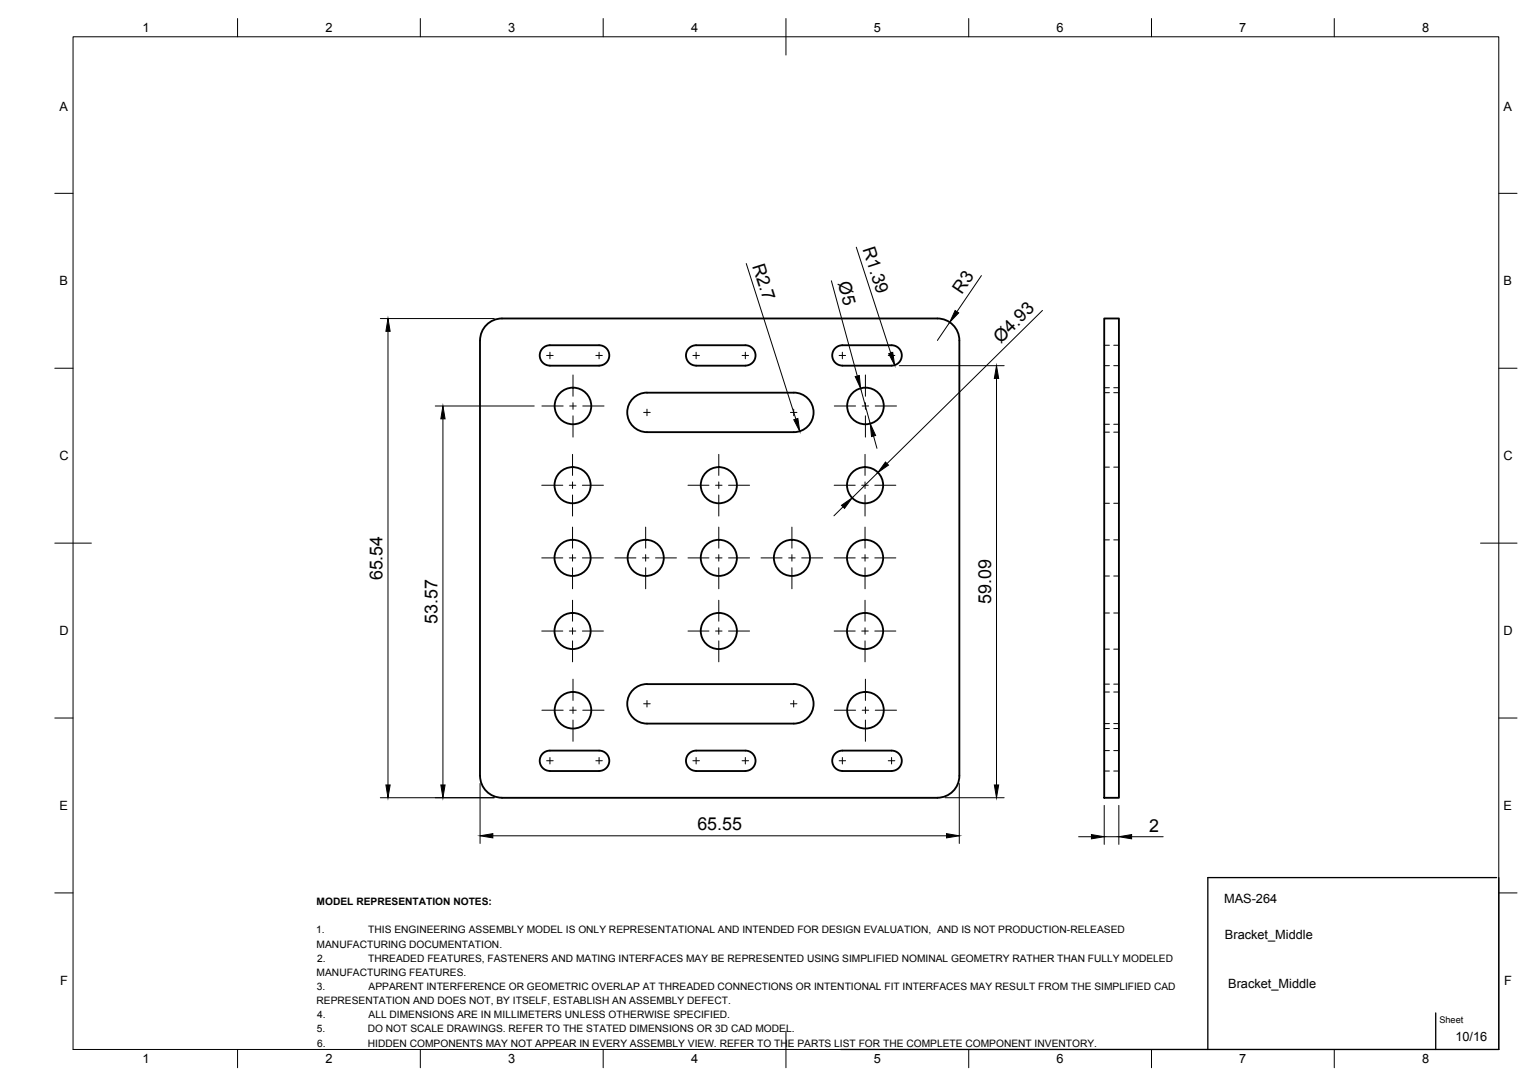
ISO-10303-21;
HEADER;
/* Generated by software containing ST-Developer
 * from STEP Tools, Inc. (www.steptools.com) 
 */

FILE_DESCRIPTION(
/* description */ (''),
/* implementation_level */ '2;1');

FILE_NAME(
/* name */ 'Bracket_Middle.step',
/* time_stamp */ '2026-10-12T15:37:13-07:00',
/* author */ (''),
/* organization */ (''),
/* preprocessor_version */ 'ST-DEVELOPER v20.2',
/* originating_system */ 'Autodesk Translation Framework v15.15.0.0',
/* authorisation */ '');

FILE_SCHEMA (('AUTOMOTIVE_DESIGN { 1 0 10303 214 3 1 1 }'));
ENDSEC;

DATA;
#10=MECHANICAL_DESIGN_GEOMETRIC_PRESENTATION_REPRESENTATION('',(#355),#36460);
#116=SHAPE_REPRESENTATION_RELATIONSHIP('SRR','None',#36528,#129);
#129=ADVANCED_BREP_SHAPE_REPRESENTATION('',(#387),#36457);
#207=FACE_BOUND('',#2295,.T.);
#208=FACE_BOUND('',#2296,.T.);
#209=FACE_BOUND('',#2297,.T.);
#210=FACE_BOUND('',#2298,.T.);
#211=FACE_BOUND('',#2299,.T.);
#212=FACE_BOUND('',#2300,.T.);
#213=FACE_BOUND('',#2301,.T.);
#214=FACE_BOUND('',#2302,.T.);
#215=FACE_BOUND('',#2303,.T.);
#216=FACE_BOUND('',#2304,.T.);
#217=FACE_BOUND('',#2305,.T.);
#218=FACE_BOUND('',#2306,.T.);
#219=FACE_BOUND('',#2307,.T.);
#220=FACE_BOUND('',#2308,.T.);
#221=FACE_BOUND('',#2309,.T.);
#222=FACE_BOUND('',#2310,.T.);
#223=FACE_BOUND('',#2311,.T.);
#224=FACE_BOUND('',#2312,.T.);
#225=FACE_BOUND('',#2313,.T.);
#226=FACE_BOUND('',#2314,.T.);
#227=FACE_BOUND('',#2315,.T.);
#228=FACE_BOUND('',#2316,.T.);
#229=FACE_BOUND('',#2317,.T.);
#230=FACE_BOUND('',#2319,.T.);
#231=FACE_BOUND('',#2320,.T.);
#232=FACE_BOUND('',#2321,.T.);
#233=FACE_BOUND('',#2322,.T.);
#234=FACE_BOUND('',#2323,.T.);
#235=FACE_BOUND('',#2324,.T.);
#236=FACE_BOUND('',#2325,.T.);
#237=FACE_BOUND('',#2326,.T.);
#238=FACE_BOUND('',#2327,.T.);
#239=FACE_BOUND('',#2328,.T.);
#240=FACE_BOUND('',#2329,.T.);
#241=FACE_BOUND('',#2330,.T.);
#242=FACE_BOUND('',#2331,.T.);
#243=FACE_BOUND('',#2332,.T.);
#244=FACE_BOUND('',#2333,.T.);
#245=FACE_BOUND('',#2334,.T.);
#246=FACE_BOUND('',#2335,.T.);
#247=FACE_BOUND('',#2336,.T.);
#248=FACE_BOUND('',#2337,.T.);
#249=FACE_BOUND('',#2338,.T.);
#250=FACE_BOUND('',#2339,.T.);
#251=FACE_BOUND('',#2340,.T.);
#252=FACE_BOUND('',#2341,.T.);
#355=STYLED_ITEM('',(#36596),#387);
#387=MANIFOLD_SOLID_BREP('Body1',#11291);
#671=PLANE('',#12235);
#672=PLANE('',#12239);
#673=PLANE('',#12258);
#674=PLANE('',#12262);
#675=PLANE('',#12266);
#676=PLANE('',#12270);
#677=PLANE('',#12289);
#678=PLANE('',#12293);
#679=PLANE('',#12303);
#680=PLANE('',#12307);
#681=PLANE('',#12311);
#682=PLANE('',#12315);
#683=PLANE('',#12319);
#684=PLANE('',#12323);
#685=PLANE('',#12327);
#686=PLANE('',#12331);
#687=PLANE('',#12341);
#688=PLANE('',#12345);
#689=PLANE('',#12349);
#690=PLANE('',#12353);
#691=PLANE('',#12357);
#692=PLANE('',#12358);
#1550=FACE_OUTER_BOUND('',#2239,.T.);
#1551=FACE_OUTER_BOUND('',#2240,.T.);
#1552=FACE_OUTER_BOUND('',#2241,.T.);
#1553=FACE_OUTER_BOUND('',#2242,.T.);
#1554=FACE_OUTER_BOUND('',#2243,.T.);
#1555=FACE_OUTER_BOUND('',#2244,.T.);
#1556=FACE_OUTER_BOUND('',#2245,.T.);
#1557=FACE_OUTER_BOUND('',#2246,.T.);
#1558=FACE_OUTER_BOUND('',#2247,.T.);
#1559=FACE_OUTER_BOUND('',#2248,.T.);
#1560=FACE_OUTER_BOUND('',#2249,.T.);
#1561=FACE_OUTER_BOUND('',#2250,.T.);
#1562=FACE_OUTER_BOUND('',#2251,.T.);
#1563=FACE_OUTER_BOUND('',#2252,.T.);
#1564=FACE_OUTER_BOUND('',#2253,.T.);
#1565=FACE_OUTER_BOUND('',#2254,.T.);
#1566=FACE_OUTER_BOUND('',#2255,.T.);
#1567=FACE_OUTER_BOUND('',#2256,.T.);
#1568=FACE_OUTER_BOUND('',#2257,.T.);
#1569=FACE_OUTER_BOUND('',#2258,.T.);
#1570=FACE_OUTER_BOUND('',#2259,.T.);
#1571=FACE_OUTER_BOUND('',#2260,.T.);
#1572=FACE_OUTER_BOUND('',#2261,.T.);
#1573=FACE_OUTER_BOUND('',#2262,.T.);
#1574=FACE_OUTER_BOUND('',#2263,.T.);
#1575=FACE_OUTER_BOUND('',#2264,.T.);
#1576=FACE_OUTER_BOUND('',#2265,.T.);
#1577=FACE_OUTER_BOUND('',#2266,.T.);
#1578=FACE_OUTER_BOUND('',#2267,.T.);
#1579=FACE_OUTER_BOUND('',#2268,.T.);
#1580=FACE_OUTER_BOUND('',#2269,.T.);
#1581=FACE_OUTER_BOUND('',#2270,.T.);
#1582=FACE_OUTER_BOUND('',#2271,.T.);
#1583=FACE_OUTER_BOUND('',#2272,.T.);
#1584=FACE_OUTER_BOUND('',#2273,.T.);
#1585=FACE_OUTER_BOUND('',#2274,.T.);
#1586=FACE_OUTER_BOUND('',#2275,.T.);
#1587=FACE_OUTER_BOUND('',#2276,.T.);
#1588=FACE_OUTER_BOUND('',#2277,.T.);
#1589=FACE_OUTER_BOUND('',#2278,.T.);
#1590=FACE_OUTER_BOUND('',#2279,.T.);
#1591=FACE_OUTER_BOUND('',#2280,.T.);
#1592=FACE_OUTER_BOUND('',#2281,.T.);
#1593=FACE_OUTER_BOUND('',#2282,.T.);
#1594=FACE_OUTER_BOUND('',#2283,.T.);
#1595=FACE_OUTER_BOUND('',#2284,.T.);
#1596=FACE_OUTER_BOUND('',#2285,.T.);
#1597=FACE_OUTER_BOUND('',#2286,.T.);
#1598=FACE_OUTER_BOUND('',#2287,.T.);
#1599=FACE_OUTER_BOUND('',#2288,.T.);
#1600=FACE_OUTER_BOUND('',#2289,.T.);
#1601=FACE_OUTER_BOUND('',#2290,.T.);
#1602=FACE_OUTER_BOUND('',#2291,.T.);
#1603=FACE_OUTER_BOUND('',#2292,.T.);
#1604=FACE_OUTER_BOUND('',#2293,.T.);
#1605=FACE_OUTER_BOUND('',#2294,.T.);
#1606=FACE_OUTER_BOUND('',#2318,.T.);
#2239=EDGE_LOOP('',(#9938,#9939,#9940,#9941));
#2240=EDGE_LOOP('',(#9942,#9943,#9944,#9945));
#2241=EDGE_LOOP('',(#9946,#9947,#9948,#9949));
#2242=EDGE_LOOP('',(#9950,#9951,#9952,#9953));
#2243=EDGE_LOOP('',(#9954,#9955,#9956,#9957));
#2244=EDGE_LOOP('',(#9958,#9959,#9960,#9961));
#2245=EDGE_LOOP('',(#9962,#9963,#9964,#9965));
#2246=EDGE_LOOP('',(#9966,#9967,#9968,#9969));
#2247=EDGE_LOOP('',(#9970,#9971,#9972,#9973));
#2248=EDGE_LOOP('',(#9974,#9975,#9976,#9977));
#2249=EDGE_LOOP('',(#9978,#9979,#9980,#9981));
#2250=EDGE_LOOP('',(#9982,#9983,#9984,#9985));
#2251=EDGE_LOOP('',(#9986,#9987,#9988,#9989));
#2252=EDGE_LOOP('',(#9990,#9991,#9992,#9993));
#2253=EDGE_LOOP('',(#9994,#9995,#9996,#9997));
#2254=EDGE_LOOP('',(#9998,#9999,#10000,#10001));
#2255=EDGE_LOOP('',(#10002,#10003,#10004,#10005));
#2256=EDGE_LOOP('',(#10006,#10007,#10008,#10009));
#2257=EDGE_LOOP('',(#10010,#10011,#10012,#10013));
#2258=EDGE_LOOP('',(#10014,#10015,#10016,#10017));
#2259=EDGE_LOOP('',(#10018,#10019,#10020,#10021));
#2260=EDGE_LOOP('',(#10022,#10023,#10024,#10025));
#2261=EDGE_LOOP('',(#10026,#10027,#10028,#10029));
#2262=EDGE_LOOP('',(#10030,#10031,#10032,#10033));
#2263=EDGE_LOOP('',(#10034,#10035,#10036,#10037));
#2264=EDGE_LOOP('',(#10038,#10039,#10040,#10041));
#2265=EDGE_LOOP('',(#10042,#10043,#10044,#10045));
#2266=EDGE_LOOP('',(#10046,#10047,#10048,#10049));
#2267=EDGE_LOOP('',(#10050,#10051,#10052,#10053));
#2268=EDGE_LOOP('',(#10054,#10055,#10056,#10057));
#2269=EDGE_LOOP('',(#10058,#10059,#10060,#10061));
#2270=EDGE_LOOP('',(#10062,#10063,#10064,#10065));
#2271=EDGE_LOOP('',(#10066,#10067,#10068,#10069));
#2272=EDGE_LOOP('',(#10070,#10071,#10072,#10073));
#2273=EDGE_LOOP('',(#10074,#10075,#10076,#10077));
#2274=EDGE_LOOP('',(#10078,#10079,#10080,#10081));
#2275=EDGE_LOOP('',(#10082,#10083,#10084,#10085));
#2276=EDGE_LOOP('',(#10086,#10087,#10088,#10089));
#2277=EDGE_LOOP('',(#10090,#10091,#10092,#10093));
#2278=EDGE_LOOP('',(#10094,#10095,#10096,#10097));
#2279=EDGE_LOOP('',(#10098,#10099,#10100,#10101));
#2280=EDGE_LOOP('',(#10102,#10103,#10104,#10105));
#2281=EDGE_LOOP('',(#10106,#10107,#10108,#10109));
#2282=EDGE_LOOP('',(#10110,#10111,#10112,#10113));
#2283=EDGE_LOOP('',(#10114,#10115,#10116,#10117));
#2284=EDGE_LOOP('',(#10118,#10119,#10120,#10121));
#2285=EDGE_LOOP('',(#10122,#10123,#10124,#10125));
#2286=EDGE_LOOP('',(#10126,#10127,#10128,#10129));
#2287=EDGE_LOOP('',(#10130,#10131,#10132,#10133));
#2288=EDGE_LOOP('',(#10134,#10135,#10136,#10137));
#2289=EDGE_LOOP('',(#10138,#10139,#10140,#10141));
#2290=EDGE_LOOP('',(#10142,#10143,#10144,#10145));
#2291=EDGE_LOOP('',(#10146,#10147,#10148,#10149));
#2292=EDGE_LOOP('',(#10150,#10151,#10152,#10153));
#2293=EDGE_LOOP('',(#10154,#10155,#10156,#10157));
#2294=EDGE_LOOP('',(#10158,#10159,#10160,#10161,#10162,#10163,#10164,#10165));
#2295=EDGE_LOOP('',(#10166));
#2296=EDGE_LOOP('',(#10167));
#2297=EDGE_LOOP('',(#10168,#10169,#10170,#10171));
#2298=EDGE_LOOP('',(#10172,#10173,#10174,#10175));
#2299=EDGE_LOOP('',(#10176,#10177,#10178,#10179));
#2300=EDGE_LOOP('',(#10180,#10181,#10182,#10183));
#2301=EDGE_LOOP('',(#10184));
#2302=EDGE_LOOP('',(#10185));
#2303=EDGE_LOOP('',(#10186,#10187,#10188,#10189));
#2304=EDGE_LOOP('',(#10190));
#2305=EDGE_LOOP('',(#10191));
#2306=EDGE_LOOP('',(#10192));
#2307=EDGE_LOOP('',(#10193));
#2308=EDGE_LOOP('',(#10194));
#2309=EDGE_LOOP('',(#10195,#10196,#10197,#10198));
#2310=EDGE_LOOP('',(#10199,#10200,#10201,#10202));
#2311=EDGE_LOOP('',(#10203));
#2312=EDGE_LOOP('',(#10204));
#2313=EDGE_LOOP('',(#10205));
#2314=EDGE_LOOP('',(#10206));
#2315=EDGE_LOOP('',(#10207));
#2316=EDGE_LOOP('',(#10208,#10209,#10210,#10211));
#2317=EDGE_LOOP('',(#10212));
#2318=EDGE_LOOP('',(#10213,#10214,#10215,#10216,#10217,#10218,#10219,#10220));
#2319=EDGE_LOOP('',(#10221));
#2320=EDGE_LOOP('',(#10222));
#2321=EDGE_LOOP('',(#10223,#10224,#10225,#10226));
#2322=EDGE_LOOP('',(#10227,#10228,#10229,#10230));
#2323=EDGE_LOOP('',(#10231,#10232,#10233,#10234));
#2324=EDGE_LOOP('',(#10235,#10236,#10237,#10238));
#2325=EDGE_LOOP('',(#10239));
#2326=EDGE_LOOP('',(#10240));
#2327=EDGE_LOOP('',(#10241,#10242,#10243,#10244));
#2328=EDGE_LOOP('',(#10245));
#2329=EDGE_LOOP('',(#10246));
#2330=EDGE_LOOP('',(#10247));
#2331=EDGE_LOOP('',(#10248));
#2332=EDGE_LOOP('',(#10249));
#2333=EDGE_LOOP('',(#10250,#10251,#10252,#10253));
#2334=EDGE_LOOP('',(#10254,#10255,#10256,#10257));
#2335=EDGE_LOOP('',(#10258));
#2336=EDGE_LOOP('',(#10259));
#2337=EDGE_LOOP('',(#10260));
#2338=EDGE_LOOP('',(#10261));
#2339=EDGE_LOOP('',(#10262));
#2340=EDGE_LOOP('',(#10263,#10264,#10265,#10266));
#2341=EDGE_LOOP('',(#10267));
#3192=LINE('',#35931,#4138);
#3193=LINE('',#35936,#4139);
#3194=LINE('',#35938,#4140);
#3195=LINE('',#35940,#4141);
#3196=LINE('',#35941,#4142);
#3197=LINE('',#35947,#4143);
#3198=LINE('',#35950,#4144);
#3199=LINE('',#35952,#4145);
#3200=LINE('',#35953,#4146);
#3201=LINE('',#35961,#4147);
#3202=LINE('',#35967,#4148);
#3203=LINE('',#35973,#4149);
#3204=LINE('',#35979,#4150);
#3205=LINE('',#35985,#4151);
#3206=LINE('',#35990,#4152);
#3207=LINE('',#35992,#4153);
#3208=LINE('',#35994,#4154);
#3209=LINE('',#35995,#4155);
#3210=LINE('',#36001,#4156);
#3211=LINE('',#36004,#4157);
#3212=LINE('',#36006,#4158);
#3213=LINE('',#36007,#4159);
#3214=LINE('',#36014,#4160);
#3215=LINE('',#36016,#4161);
#3216=LINE('',#36018,#4162);
#3217=LINE('',#36019,#4163);
#3218=LINE('',#36025,#4164);
#3219=LINE('',#36028,#4165);
#3220=LINE('',#36030,#4166);
#3221=LINE('',#36031,#4167);
#3222=LINE('',#36039,#4168);
#3223=LINE('',#36045,#4169);
#3224=LINE('',#36051,#4170);
#3225=LINE('',#36057,#4171);
#3226=LINE('',#36063,#4172);
#3227=LINE('',#36068,#4173);
#3228=LINE('',#36070,#4174);
#3229=LINE('',#36072,#4175);
#3230=LINE('',#36073,#4176);
#3231=LINE('',#36079,#4177);
#3232=LINE('',#36082,#4178);
#3233=LINE('',#36084,#4179);
#3234=LINE('',#36085,#4180);
#3235=LINE('',#36093,#4181);
#3236=LINE('',#36099,#4182);
#3237=LINE('',#36104,#4183);
#3238=LINE('',#36106,#4184);
#3239=LINE('',#36108,#4185);
#3240=LINE('',#36109,#4186);
#3241=LINE('',#36115,#4187);
#3242=LINE('',#36118,#4188);
#3243=LINE('',#36120,#4189);
#3244=LINE('',#36121,#4190);
#3245=LINE('',#36128,#4191);
#3246=LINE('',#36130,#4192);
#3247=LINE('',#36132,#4193);
#3248=LINE('',#36133,#4194);
#3249=LINE('',#36139,#4195);
#3250=LINE('',#36142,#4196);
#3251=LINE('',#36144,#4197);
#3252=LINE('',#36145,#4198);
#3253=LINE('',#36152,#4199);
#3254=LINE('',#36154,#4200);
#3255=LINE('',#36156,#4201);
#3256=LINE('',#36157,#4202);
#3257=LINE('',#36163,#4203);
#3258=LINE('',#36166,#4204);
#3259=LINE('',#36168,#4205);
#3260=LINE('',#36169,#4206);
#3261=LINE('',#36176,#4207);
#3262=LINE('',#36178,#4208);
#3263=LINE('',#36180,#4209);
#3264=LINE('',#36181,#4210);
#3265=LINE('',#36187,#4211);
#3266=LINE('',#36190,#4212);
#3267=LINE('',#36192,#4213);
#3268=LINE('',#36193,#4214);
#3269=LINE('',#36201,#4215);
#3270=LINE('',#36207,#4216);
#3271=LINE('',#36212,#4217);
#3272=LINE('',#36214,#4218);
#3273=LINE('',#36216,#4219);
#3274=LINE('',#36217,#4220);
#3275=LINE('',#36223,#4221);
#3276=LINE('',#36226,#4222);
#3277=LINE('',#36228,#4223);
#3278=LINE('',#36229,#4224);
#3279=LINE('',#36235,#4225);
#3280=LINE('',#36238,#4226);
#3281=LINE('',#36240,#4227);
#3282=LINE('',#36241,#4228);
#3283=LINE('',#36247,#4229);
#3284=LINE('',#36250,#4230);
#3285=LINE('',#36252,#4231);
#3286=LINE('',#36253,#4232);
#4138=VECTOR('',#14833,2.5);
#4139=VECTOR('',#14838,10.);
#4140=VECTOR('',#14839,10.);
#4141=VECTOR('',#14840,10.);
#4142=VECTOR('',#14841,10.);
#4143=VECTOR('',#14848,10.);
#4144=VECTOR('',#14851,10.);
#4145=VECTOR('',#14852,10.);
#4146=VECTOR('',#14853,10.);
#4147=VECTOR('',#14864,2.46675107308807);
#4148=VECTOR('',#14871,2.46675107308807);
#4149=VECTOR('',#14878,2.46675107308807);
#4150=VECTOR('',#14885,2.46675107308807);
#4151=VECTOR('',#14892,2.46675107308807);
#4152=VECTOR('',#14897,10.);
#4153=VECTOR('',#14898,10.);
#4154=VECTOR('',#14899,10.);
#4155=VECTOR('',#14900,10.);
#4156=VECTOR('',#14907,10.);
#4157=VECTOR('',#14910,10.);
#4158=VECTOR('',#14911,10.);
#4159=VECTOR('',#14912,10.);
#4160=VECTOR('',#14921,10.);
#4161=VECTOR('',#14922,10.);
#4162=VECTOR('',#14923,10.);
#4163=VECTOR('',#14924,10.);
#4164=VECTOR('',#14931,10.);
#4165=VECTOR('',#14934,10.);
#4166=VECTOR('',#14935,10.);
#4167=VECTOR('',#14936,10.);
#4168=VECTOR('',#14947,2.5);
#4169=VECTOR('',#14954,2.46675107308807);
#4170=VECTOR('',#14961,2.5);
#4171=VECTOR('',#14968,2.46675107308807);
#4172=VECTOR('',#14975,2.46675107308807);
#4173=VECTOR('',#14980,10.);
#4174=VECTOR('',#14981,10.);
#4175=VECTOR('',#14982,10.);
#4176=VECTOR('',#14983,10.);
#4177=VECTOR('',#14990,10.);
#4178=VECTOR('',#14993,10.);
#4179=VECTOR('',#14994,10.);
#4180=VECTOR('',#14995,10.);
#4181=VECTOR('',#15006,2.5);
#4182=VECTOR('',#15013,2.46675107308807);
#4183=VECTOR('',#15018,10.);
#4184=VECTOR('',#15019,10.);
#4185=VECTOR('',#15020,10.);
#4186=VECTOR('',#15021,10.);
#4187=VECTOR('',#15028,10.);
#4188=VECTOR('',#15031,10.);
#4189=VECTOR('',#15032,10.);
#4190=VECTOR('',#15033,10.);
#4191=VECTOR('',#15042,10.);
#4192=VECTOR('',#15043,10.);
#4193=VECTOR('',#15044,10.);
#4194=VECTOR('',#15045,10.);
#4195=VECTOR('',#15052,10.);
#4196=VECTOR('',#15055,10.);
#4197=VECTOR('',#15056,10.);
#4198=VECTOR('',#15057,10.);
#4199=VECTOR('',#15066,10.);
#4200=VECTOR('',#15067,10.);
#4201=VECTOR('',#15068,10.);
#4202=VECTOR('',#15069,10.);
#4203=VECTOR('',#15076,10.);
#4204=VECTOR('',#15079,10.);
#4205=VECTOR('',#15080,10.);
#4206=VECTOR('',#15081,10.);
#4207=VECTOR('',#15090,10.);
#4208=VECTOR('',#15091,10.);
#4209=VECTOR('',#15092,10.);
#4210=VECTOR('',#15093,10.);
#4211=VECTOR('',#15100,10.);
#4212=VECTOR('',#15103,10.);
#4213=VECTOR('',#15104,10.);
#4214=VECTOR('',#15105,10.);
#4215=VECTOR('',#15116,2.46675107308807);
#4216=VECTOR('',#15123,2.46675107308807);
#4217=VECTOR('',#15128,10.);
#4218=VECTOR('',#15129,10.);
#4219=VECTOR('',#15130,10.);
#4220=VECTOR('',#15131,10.);
#4221=VECTOR('',#15138,10.);
#4222=VECTOR('',#15141,10.);
#4223=VECTOR('',#15142,10.);
#4224=VECTOR('',#15143,10.);
#4225=VECTOR('',#15150,10.);
#4226=VECTOR('',#15153,10.);
#4227=VECTOR('',#15154,10.);
#4228=VECTOR('',#15155,10.);
#4229=VECTOR('',#15162,10.);
#4230=VECTOR('',#15165,10.);
#4231=VECTOR('',#15166,10.);
#4232=VECTOR('',#15167,10.);
#4497=CIRCLE('',#12233,2.5);
#4498=CIRCLE('',#12234,2.5);
#4499=CIRCLE('',#12237,1.3925055570925);
#4500=CIRCLE('',#12238,1.3925055570925);
#4501=CIRCLE('',#12241,1.3925055570925);
#4502=CIRCLE('',#12242,1.3925055570925);
#4503=CIRCLE('',#12244,2.46675107308807);
#4504=CIRCLE('',#12245,2.46675107308807);
#4505=CIRCLE('',#12247,2.46675107308807);
#4506=CIRCLE('',#12248,2.46675107308807);
#4507=CIRCLE('',#12250,2.46675107308807);
#4508=CIRCLE('',#12251,2.46675107308807);
#4509=CIRCLE('',#12253,2.46675107308807);
#4510=CIRCLE('',#12254,2.46675107308807);
#4511=CIRCLE('',#12256,2.46675107308807);
#4512=CIRCLE('',#12257,2.46675107308807);
#4513=CIRCLE('',#12260,2.69990459756453);
#4514=CIRCLE('',#12261,2.69990459756453);
#4515=CIRCLE('',#12264,2.69990459756453);
#4516=CIRCLE('',#12265,2.69990459756453);
#4517=CIRCLE('',#12268,1.3925055570925);
#4518=CIRCLE('',#12269,1.3925055570925);
#4519=CIRCLE('',#12272,1.3925055570925);
#4520=CIRCLE('',#12273,1.3925055570925);
#4521=CIRCLE('',#12275,2.5);
#4522=CIRCLE('',#12276,2.5);
#4523=CIRCLE('',#12278,2.46675107308807);
#4524=CIRCLE('',#12279,2.46675107308807);
#4525=CIRCLE('',#12281,2.5);
#4526=CIRCLE('',#12282,2.5);
#4527=CIRCLE('',#12284,2.46675107308807);
#4528=CIRCLE('',#12285,2.46675107308807);
#4529=CIRCLE('',#12287,2.46675107308807);
#4530=CIRCLE('',#12288,2.46675107308807);
#4531=CIRCLE('',#12291,1.3925055570925);
#4532=CIRCLE('',#12292,1.3925055570925);
#4533=CIRCLE('',#12295,1.3925055570925);
#4534=CIRCLE('',#12296,1.3925055570925);
#4535=CIRCLE('',#12298,2.5);
#4536=CIRCLE('',#12299,2.5);
#4537=CIRCLE('',#12301,2.46675107308807);
#4538=CIRCLE('',#12302,2.46675107308807);
#4539=CIRCLE('',#12305,1.3925055570925);
#4540=CIRCLE('',#12306,1.3925055570925);
#4541=CIRCLE('',#12309,1.3925055570925);
#4542=CIRCLE('',#12310,1.3925055570925);
#4543=CIRCLE('',#12313,1.3925055570925);
#4544=CIRCLE('',#12314,1.3925055570925);
#4545=CIRCLE('',#12317,1.3925055570925);
#4546=CIRCLE('',#12318,1.3925055570925);
#4547=CIRCLE('',#12321,1.3925055570925);
#4548=CIRCLE('',#12322,1.3925055570925);
#4549=CIRCLE('',#12325,1.3925055570925);
#4550=CIRCLE('',#12326,1.3925055570925);
#4551=CIRCLE('',#12329,2.69990459756453);
#4552=CIRCLE('',#12330,2.69990459756453);
#4553=CIRCLE('',#12333,2.69990459756453);
#4554=CIRCLE('',#12334,2.69990459756453);
#4555=CIRCLE('',#12336,2.46675107308807);
#4556=CIRCLE('',#12337,2.46675107308807);
#4557=CIRCLE('',#12339,2.46675107308807);
#4558=CIRCLE('',#12340,2.46675107308807);
#4559=CIRCLE('',#12343,3.00000000000004);
#4560=CIRCLE('',#12344,3.00000000000004);
#4561=CIRCLE('',#12347,3.00000000000003);
#4562=CIRCLE('',#12348,3.00000000000003);
#4563=CIRCLE('',#12351,3.00000000000004);
#4564=CIRCLE('',#12352,3.00000000000004);
#4565=CIRCLE('',#12355,3.00000000000004);
#4566=CIRCLE('',#12356,3.00000000000004);
#5495=VERTEX_POINT('',#35928);
#5496=VERTEX_POINT('',#35930);
#5497=VERTEX_POINT('',#35934);
#5498=VERTEX_POINT('',#35935);
#5499=VERTEX_POINT('',#35937);
#5500=VERTEX_POINT('',#35939);
#5501=VERTEX_POINT('',#35943);
#5502=VERTEX_POINT('',#35945);
#5503=VERTEX_POINT('',#35949);
#5504=VERTEX_POINT('',#35951);
#5505=VERTEX_POINT('',#35958);
#5506=VERTEX_POINT('',#35960);
#5507=VERTEX_POINT('',#35964);
#5508=VERTEX_POINT('',#35966);
#5509=VERTEX_POINT('',#35970);
#5510=VERTEX_POINT('',#35972);
#5511=VERTEX_POINT('',#35976);
#5512=VERTEX_POINT('',#35978);
#5513=VERTEX_POINT('',#35982);
#5514=VERTEX_POINT('',#35984);
#5515=VERTEX_POINT('',#35988);
#5516=VERTEX_POINT('',#35989);
#5517=VERTEX_POINT('',#35991);
#5518=VERTEX_POINT('',#35993);
#5519=VERTEX_POINT('',#35997);
#5520=VERTEX_POINT('',#35999);
#5521=VERTEX_POINT('',#36003);
#5522=VERTEX_POINT('',#36005);
#5523=VERTEX_POINT('',#36012);
#5524=VERTEX_POINT('',#36013);
#5525=VERTEX_POINT('',#36015);
#5526=VERTEX_POINT('',#36017);
#5527=VERTEX_POINT('',#36021);
#5528=VERTEX_POINT('',#36023);
#5529=VERTEX_POINT('',#36027);
#5530=VERTEX_POINT('',#36029);
#5531=VERTEX_POINT('',#36036);
#5532=VERTEX_POINT('',#36038);
#5533=VERTEX_POINT('',#36042);
#5534=VERTEX_POINT('',#36044);
#5535=VERTEX_POINT('',#36048);
#5536=VERTEX_POINT('',#36050);
#5537=VERTEX_POINT('',#36054);
#5538=VERTEX_POINT('',#36056);
#5539=VERTEX_POINT('',#36060);
#5540=VERTEX_POINT('',#36062);
#5541=VERTEX_POINT('',#36066);
#5542=VERTEX_POINT('',#36067);
#5543=VERTEX_POINT('',#36069);
#5544=VERTEX_POINT('',#36071);
#5545=VERTEX_POINT('',#36075);
#5546=VERTEX_POINT('',#36077);
#5547=VERTEX_POINT('',#36081);
#5548=VERTEX_POINT('',#36083);
#5549=VERTEX_POINT('',#36090);
#5550=VERTEX_POINT('',#36092);
#5551=VERTEX_POINT('',#36096);
#5552=VERTEX_POINT('',#36098);
#5553=VERTEX_POINT('',#36102);
#5554=VERTEX_POINT('',#36103);
#5555=VERTEX_POINT('',#36105);
#5556=VERTEX_POINT('',#36107);
#5557=VERTEX_POINT('',#36111);
#5558=VERTEX_POINT('',#36113);
#5559=VERTEX_POINT('',#36117);
#5560=VERTEX_POINT('',#36119);
#5561=VERTEX_POINT('',#36126);
#5562=VERTEX_POINT('',#36127);
#5563=VERTEX_POINT('',#36129);
#5564=VERTEX_POINT('',#36131);
#5565=VERTEX_POINT('',#36135);
#5566=VERTEX_POINT('',#36137);
#5567=VERTEX_POINT('',#36141);
#5568=VERTEX_POINT('',#36143);
#5569=VERTEX_POINT('',#36150);
#5570=VERTEX_POINT('',#36151);
#5571=VERTEX_POINT('',#36153);
#5572=VERTEX_POINT('',#36155);
#5573=VERTEX_POINT('',#36159);
#5574=VERTEX_POINT('',#36161);
#5575=VERTEX_POINT('',#36165);
#5576=VERTEX_POINT('',#36167);
#5577=VERTEX_POINT('',#36174);
#5578=VERTEX_POINT('',#36175);
#5579=VERTEX_POINT('',#36177);
#5580=VERTEX_POINT('',#36179);
#5581=VERTEX_POINT('',#36183);
#5582=VERTEX_POINT('',#36185);
#5583=VERTEX_POINT('',#36189);
#5584=VERTEX_POINT('',#36191);
#5585=VERTEX_POINT('',#36198);
#5586=VERTEX_POINT('',#36200);
#5587=VERTEX_POINT('',#36204);
#5588=VERTEX_POINT('',#36206);
#5589=VERTEX_POINT('',#36210);
#5590=VERTEX_POINT('',#36211);
#5591=VERTEX_POINT('',#36213);
#5592=VERTEX_POINT('',#36215);
#5593=VERTEX_POINT('',#36219);
#5594=VERTEX_POINT('',#36221);
#5595=VERTEX_POINT('',#36225);
#5596=VERTEX_POINT('',#36227);
#5597=VERTEX_POINT('',#36231);
#5598=VERTEX_POINT('',#36233);
#5599=VERTEX_POINT('',#36237);
#5600=VERTEX_POINT('',#36239);
#5601=VERTEX_POINT('',#36243);
#5602=VERTEX_POINT('',#36245);
#5603=VERTEX_POINT('',#36249);
#5604=VERTEX_POINT('',#36251);
#7000=EDGE_CURVE('',#5495,#5495,#4497,.T.);
#7001=EDGE_CURVE('',#5495,#5496,#3192,.T.);
#7002=EDGE_CURVE('',#5496,#5496,#4498,.T.);
#7003=EDGE_CURVE('',#5497,#5498,#3193,.T.);
#7004=EDGE_CURVE('',#5498,#5499,#3194,.T.);
#7005=EDGE_CURVE('',#5500,#5499,#3195,.T.);
#7006=EDGE_CURVE('',#5497,#5500,#3196,.T.);
#7007=EDGE_CURVE('',#5501,#5497,#4499,.T.);
#7008=EDGE_CURVE('',#5502,#5500,#4500,.T.);
#7009=EDGE_CURVE('',#5501,#5502,#3197,.T.);
#7010=EDGE_CURVE('',#5503,#5501,#3198,.T.);
#7011=EDGE_CURVE('',#5504,#5502,#3199,.T.);
#7012=EDGE_CURVE('',#5503,#5504,#3200,.T.);
#7013=EDGE_CURVE('',#5498,#5503,#4501,.T.);
#7014=EDGE_CURVE('',#5499,#5504,#4502,.T.);
#7015=EDGE_CURVE('',#5505,#5505,#4503,.T.);
#7016=EDGE_CURVE('',#5505,#5506,#3201,.T.);
#7017=EDGE_CURVE('',#5506,#5506,#4504,.T.);
#7018=EDGE_CURVE('',#5507,#5507,#4505,.T.);
#7019=EDGE_CURVE('',#5507,#5508,#3202,.T.);
#7020=EDGE_CURVE('',#5508,#5508,#4506,.T.);
#7021=EDGE_CURVE('',#5509,#5509,#4507,.T.);
#7022=EDGE_CURVE('',#5509,#5510,#3203,.T.);
#7023=EDGE_CURVE('',#5510,#5510,#4508,.T.);
#7024=EDGE_CURVE('',#5511,#5511,#4509,.T.);
#7025=EDGE_CURVE('',#5511,#5512,#3204,.T.);
#7026=EDGE_CURVE('',#5512,#5512,#4510,.T.);
#7027=EDGE_CURVE('',#5513,#5513,#4511,.T.);
#7028=EDGE_CURVE('',#5513,#5514,#3205,.T.);
#7029=EDGE_CURVE('',#5514,#5514,#4512,.T.);
#7030=EDGE_CURVE('',#5515,#5516,#3206,.T.);
#7031=EDGE_CURVE('',#5516,#5517,#3207,.T.);
#7032=EDGE_CURVE('',#5518,#5517,#3208,.T.);
#7033=EDGE_CURVE('',#5515,#5518,#3209,.T.);
#7034=EDGE_CURVE('',#5519,#5515,#4513,.T.);
#7035=EDGE_CURVE('',#5520,#5518,#4514,.T.);
#7036=EDGE_CURVE('',#5519,#5520,#3210,.T.);
#7037=EDGE_CURVE('',#5521,#5519,#3211,.T.);
#7038=EDGE_CURVE('',#5522,#5520,#3212,.T.);
#7039=EDGE_CURVE('',#5521,#5522,#3213,.T.);
#7040=EDGE_CURVE('',#5516,#5521,#4515,.T.);
#7041=EDGE_CURVE('',#5517,#5522,#4516,.T.);
#7042=EDGE_CURVE('',#5523,#5524,#3214,.T.);
#7043=EDGE_CURVE('',#5524,#5525,#3215,.T.);
#7044=EDGE_CURVE('',#5526,#5525,#3216,.T.);
#7045=EDGE_CURVE('',#5523,#5526,#3217,.T.);
#7046=EDGE_CURVE('',#5527,#5523,#4517,.T.);
#7047=EDGE_CURVE('',#5528,#5526,#4518,.T.);
#7048=EDGE_CURVE('',#5527,#5528,#3218,.T.);
#7049=EDGE_CURVE('',#5529,#5527,#3219,.T.);
#7050=EDGE_CURVE('',#5530,#5528,#3220,.T.);
#7051=EDGE_CURVE('',#5529,#5530,#3221,.T.);
#7052=EDGE_CURVE('',#5524,#5529,#4519,.T.);
#7053=EDGE_CURVE('',#5525,#5530,#4520,.T.);
#7054=EDGE_CURVE('',#5531,#5531,#4521,.T.);
#7055=EDGE_CURVE('',#5531,#5532,#3222,.T.);
#7056=EDGE_CURVE('',#5532,#5532,#4522,.T.);
#7057=EDGE_CURVE('',#5533,#5533,#4523,.T.);
#7058=EDGE_CURVE('',#5533,#5534,#3223,.T.);
#7059=EDGE_CURVE('',#5534,#5534,#4524,.T.);
#7060=EDGE_CURVE('',#5535,#5535,#4525,.T.);
#7061=EDGE_CURVE('',#5535,#5536,#3224,.T.);
#7062=EDGE_CURVE('',#5536,#5536,#4526,.T.);
#7063=EDGE_CURVE('',#5537,#5537,#4527,.T.);
#7064=EDGE_CURVE('',#5537,#5538,#3225,.T.);
#7065=EDGE_CURVE('',#5538,#5538,#4528,.T.);
#7066=EDGE_CURVE('',#5539,#5539,#4529,.T.);
#7067=EDGE_CURVE('',#5539,#5540,#3226,.T.);
#7068=EDGE_CURVE('',#5540,#5540,#4530,.T.);
#7069=EDGE_CURVE('',#5541,#5542,#3227,.T.);
#7070=EDGE_CURVE('',#5542,#5543,#3228,.T.);
#7071=EDGE_CURVE('',#5544,#5543,#3229,.T.);
#7072=EDGE_CURVE('',#5541,#5544,#3230,.T.);
#7073=EDGE_CURVE('',#5545,#5541,#4531,.T.);
#7074=EDGE_CURVE('',#5546,#5544,#4532,.T.);
#7075=EDGE_CURVE('',#5545,#5546,#3231,.T.);
#7076=EDGE_CURVE('',#5547,#5545,#3232,.T.);
#7077=EDGE_CURVE('',#5548,#5546,#3233,.T.);
#7078=EDGE_CURVE('',#5547,#5548,#3234,.T.);
#7079=EDGE_CURVE('',#5542,#5547,#4533,.T.);
#7080=EDGE_CURVE('',#5543,#5548,#4534,.T.);
#7081=EDGE_CURVE('',#5549,#5549,#4535,.T.);
#7082=EDGE_CURVE('',#5549,#5550,#3235,.T.);
#7083=EDGE_CURVE('',#5550,#5550,#4536,.T.);
#7084=EDGE_CURVE('',#5551,#5551,#4537,.T.);
#7085=EDGE_CURVE('',#5551,#5552,#3236,.T.);
#7086=EDGE_CURVE('',#5552,#5552,#4538,.T.);
#7087=EDGE_CURVE('',#5553,#5554,#3237,.T.);
#7088=EDGE_CURVE('',#5554,#5555,#3238,.T.);
#7089=EDGE_CURVE('',#5556,#5555,#3239,.T.);
#7090=EDGE_CURVE('',#5553,#5556,#3240,.T.);
#7091=EDGE_CURVE('',#5557,#5553,#4539,.T.);
#7092=EDGE_CURVE('',#5558,#5556,#4540,.T.);
#7093=EDGE_CURVE('',#5557,#5558,#3241,.T.);
#7094=EDGE_CURVE('',#5559,#5557,#3242,.T.);
#7095=EDGE_CURVE('',#5560,#5558,#3243,.T.);
#7096=EDGE_CURVE('',#5559,#5560,#3244,.T.);
#7097=EDGE_CURVE('',#5554,#5559,#4541,.T.);
#7098=EDGE_CURVE('',#5555,#5560,#4542,.T.);
#7099=EDGE_CURVE('',#5561,#5562,#3245,.T.);
#7100=EDGE_CURVE('',#5562,#5563,#3246,.T.);
#7101=EDGE_CURVE('',#5564,#5563,#3247,.T.);
#7102=EDGE_CURVE('',#5561,#5564,#3248,.T.);
#7103=EDGE_CURVE('',#5565,#5561,#4543,.T.);
#7104=EDGE_CURVE('',#5566,#5564,#4544,.T.);
#7105=EDGE_CURVE('',#5565,#5566,#3249,.T.);
#7106=EDGE_CURVE('',#5567,#5565,#3250,.T.);
#7107=EDGE_CURVE('',#5568,#5566,#3251,.T.);
#7108=EDGE_CURVE('',#5567,#5568,#3252,.T.);
#7109=EDGE_CURVE('',#5562,#5567,#4545,.T.);
#7110=EDGE_CURVE('',#5563,#5568,#4546,.T.);
#7111=EDGE_CURVE('',#5569,#5570,#3253,.T.);
#7112=EDGE_CURVE('',#5570,#5571,#3254,.T.);
#7113=EDGE_CURVE('',#5572,#5571,#3255,.T.);
#7114=EDGE_CURVE('',#5569,#5572,#3256,.T.);
#7115=EDGE_CURVE('',#5573,#5569,#4547,.T.);
#7116=EDGE_CURVE('',#5574,#5572,#4548,.T.);
#7117=EDGE_CURVE('',#5573,#5574,#3257,.T.);
#7118=EDGE_CURVE('',#5575,#5573,#3258,.T.);
#7119=EDGE_CURVE('',#5576,#5574,#3259,.T.);
#7120=EDGE_CURVE('',#5575,#5576,#3260,.T.);
#7121=EDGE_CURVE('',#5570,#5575,#4549,.T.);
#7122=EDGE_CURVE('',#5571,#5576,#4550,.T.);
#7123=EDGE_CURVE('',#5577,#5578,#3261,.T.);
#7124=EDGE_CURVE('',#5578,#5579,#3262,.T.);
#7125=EDGE_CURVE('',#5580,#5579,#3263,.T.);
#7126=EDGE_CURVE('',#5577,#5580,#3264,.T.);
#7127=EDGE_CURVE('',#5581,#5577,#4551,.T.);
#7128=EDGE_CURVE('',#5582,#5580,#4552,.T.);
#7129=EDGE_CURVE('',#5581,#5582,#3265,.T.);
#7130=EDGE_CURVE('',#5583,#5581,#3266,.T.);
#7131=EDGE_CURVE('',#5584,#5582,#3267,.T.);
#7132=EDGE_CURVE('',#5583,#5584,#3268,.T.);
#7133=EDGE_CURVE('',#5578,#5583,#4553,.T.);
#7134=EDGE_CURVE('',#5579,#5584,#4554,.T.);
#7135=EDGE_CURVE('',#5585,#5585,#4555,.T.);
#7136=EDGE_CURVE('',#5585,#5586,#3269,.T.);
#7137=EDGE_CURVE('',#5586,#5586,#4556,.T.);
#7138=EDGE_CURVE('',#5587,#5587,#4557,.T.);
#7139=EDGE_CURVE('',#5587,#5588,#3270,.T.);
#7140=EDGE_CURVE('',#5588,#5588,#4558,.T.);
#7141=EDGE_CURVE('',#5589,#5590,#3271,.T.);
#7142=EDGE_CURVE('',#5589,#5591,#3272,.T.);
#7143=EDGE_CURVE('',#5592,#5591,#3273,.T.);
#7144=EDGE_CURVE('',#5590,#5592,#3274,.T.);
#7145=EDGE_CURVE('',#5593,#5590,#4559,.T.);
#7146=EDGE_CURVE('',#5594,#5592,#4560,.T.);
#7147=EDGE_CURVE('',#5593,#5594,#3275,.T.);
#7148=EDGE_CURVE('',#5593,#5595,#3276,.T.);
#7149=EDGE_CURVE('',#5596,#5594,#3277,.T.);
#7150=EDGE_CURVE('',#5595,#5596,#3278,.T.);
#7151=EDGE_CURVE('',#5597,#5595,#4561,.T.);
#7152=EDGE_CURVE('',#5598,#5596,#4562,.T.);
#7153=EDGE_CURVE('',#5597,#5598,#3279,.T.);
#7154=EDGE_CURVE('',#5597,#5599,#3280,.T.);
#7155=EDGE_CURVE('',#5600,#5598,#3281,.T.);
#7156=EDGE_CURVE('',#5599,#5600,#3282,.T.);
#7157=EDGE_CURVE('',#5601,#5599,#4563,.T.);
#7158=EDGE_CURVE('',#5602,#5600,#4564,.T.);
#7159=EDGE_CURVE('',#5601,#5602,#3283,.T.);
#7160=EDGE_CURVE('',#5601,#5603,#3284,.T.);
#7161=EDGE_CURVE('',#5604,#5602,#3285,.T.);
#7162=EDGE_CURVE('',#5603,#5604,#3286,.T.);
#7163=EDGE_CURVE('',#5589,#5603,#4565,.T.);
#7164=EDGE_CURVE('',#5591,#5604,#4566,.T.);
#9938=ORIENTED_EDGE('',*,*,#7000,.T.);
#9939=ORIENTED_EDGE('',*,*,#7001,.T.);
#9940=ORIENTED_EDGE('',*,*,#7002,.F.);
#9941=ORIENTED_EDGE('',*,*,#7001,.F.);
#9942=ORIENTED_EDGE('',*,*,#7003,.T.);
#9943=ORIENTED_EDGE('',*,*,#7004,.T.);
#9944=ORIENTED_EDGE('',*,*,#7005,.F.);
#9945=ORIENTED_EDGE('',*,*,#7006,.F.);
#9946=ORIENTED_EDGE('',*,*,#7007,.T.);
#9947=ORIENTED_EDGE('',*,*,#7006,.T.);
#9948=ORIENTED_EDGE('',*,*,#7008,.F.);
#9949=ORIENTED_EDGE('',*,*,#7009,.F.);
#9950=ORIENTED_EDGE('',*,*,#7010,.T.);
#9951=ORIENTED_EDGE('',*,*,#7009,.T.);
#9952=ORIENTED_EDGE('',*,*,#7011,.F.);
#9953=ORIENTED_EDGE('',*,*,#7012,.F.);
#9954=ORIENTED_EDGE('',*,*,#7013,.T.);
#9955=ORIENTED_EDGE('',*,*,#7012,.T.);
#9956=ORIENTED_EDGE('',*,*,#7014,.F.);
#9957=ORIENTED_EDGE('',*,*,#7004,.F.);
#9958=ORIENTED_EDGE('',*,*,#7015,.T.);
#9959=ORIENTED_EDGE('',*,*,#7016,.T.);
#9960=ORIENTED_EDGE('',*,*,#7017,.F.);
#9961=ORIENTED_EDGE('',*,*,#7016,.F.);
#9962=ORIENTED_EDGE('',*,*,#7018,.T.);
#9963=ORIENTED_EDGE('',*,*,#7019,.T.);
#9964=ORIENTED_EDGE('',*,*,#7020,.F.);
#9965=ORIENTED_EDGE('',*,*,#7019,.F.);
#9966=ORIENTED_EDGE('',*,*,#7021,.T.);
#9967=ORIENTED_EDGE('',*,*,#7022,.T.);
#9968=ORIENTED_EDGE('',*,*,#7023,.F.);
#9969=ORIENTED_EDGE('',*,*,#7022,.F.);
#9970=ORIENTED_EDGE('',*,*,#7024,.T.);
#9971=ORIENTED_EDGE('',*,*,#7025,.T.);
#9972=ORIENTED_EDGE('',*,*,#7026,.F.);
#9973=ORIENTED_EDGE('',*,*,#7025,.F.);
#9974=ORIENTED_EDGE('',*,*,#7027,.T.);
#9975=ORIENTED_EDGE('',*,*,#7028,.T.);
#9976=ORIENTED_EDGE('',*,*,#7029,.F.);
#9977=ORIENTED_EDGE('',*,*,#7028,.F.);
#9978=ORIENTED_EDGE('',*,*,#7030,.T.);
#9979=ORIENTED_EDGE('',*,*,#7031,.T.);
#9980=ORIENTED_EDGE('',*,*,#7032,.F.);
#9981=ORIENTED_EDGE('',*,*,#7033,.F.);
#9982=ORIENTED_EDGE('',*,*,#7034,.T.);
#9983=ORIENTED_EDGE('',*,*,#7033,.T.);
#9984=ORIENTED_EDGE('',*,*,#7035,.F.);
#9985=ORIENTED_EDGE('',*,*,#7036,.F.);
#9986=ORIENTED_EDGE('',*,*,#7037,.T.);
#9987=ORIENTED_EDGE('',*,*,#7036,.T.);
#9988=ORIENTED_EDGE('',*,*,#7038,.F.);
#9989=ORIENTED_EDGE('',*,*,#7039,.F.);
#9990=ORIENTED_EDGE('',*,*,#7040,.T.);
#9991=ORIENTED_EDGE('',*,*,#7039,.T.);
#9992=ORIENTED_EDGE('',*,*,#7041,.F.);
#9993=ORIENTED_EDGE('',*,*,#7031,.F.);
#9994=ORIENTED_EDGE('',*,*,#7042,.T.);
#9995=ORIENTED_EDGE('',*,*,#7043,.T.);
#9996=ORIENTED_EDGE('',*,*,#7044,.F.);
#9997=ORIENTED_EDGE('',*,*,#7045,.F.);
#9998=ORIENTED_EDGE('',*,*,#7046,.T.);
#9999=ORIENTED_EDGE('',*,*,#7045,.T.);
#10000=ORIENTED_EDGE('',*,*,#7047,.F.);
#10001=ORIENTED_EDGE('',*,*,#7048,.F.);
#10002=ORIENTED_EDGE('',*,*,#7049,.T.);
#10003=ORIENTED_EDGE('',*,*,#7048,.T.);
#10004=ORIENTED_EDGE('',*,*,#7050,.F.);
#10005=ORIENTED_EDGE('',*,*,#7051,.F.);
#10006=ORIENTED_EDGE('',*,*,#7052,.T.);
#10007=ORIENTED_EDGE('',*,*,#7051,.T.);
#10008=ORIENTED_EDGE('',*,*,#7053,.F.);
#10009=ORIENTED_EDGE('',*,*,#7043,.F.);
#10010=ORIENTED_EDGE('',*,*,#7054,.T.);
#10011=ORIENTED_EDGE('',*,*,#7055,.T.);
#10012=ORIENTED_EDGE('',*,*,#7056,.F.);
#10013=ORIENTED_EDGE('',*,*,#7055,.F.);
#10014=ORIENTED_EDGE('',*,*,#7057,.T.);
#10015=ORIENTED_EDGE('',*,*,#7058,.T.);
#10016=ORIENTED_EDGE('',*,*,#7059,.F.);
#10017=ORIENTED_EDGE('',*,*,#7058,.F.);
#10018=ORIENTED_EDGE('',*,*,#7060,.T.);
#10019=ORIENTED_EDGE('',*,*,#7061,.T.);
#10020=ORIENTED_EDGE('',*,*,#7062,.F.);
#10021=ORIENTED_EDGE('',*,*,#7061,.F.);
#10022=ORIENTED_EDGE('',*,*,#7063,.T.);
#10023=ORIENTED_EDGE('',*,*,#7064,.T.);
#10024=ORIENTED_EDGE('',*,*,#7065,.F.);
#10025=ORIENTED_EDGE('',*,*,#7064,.F.);
#10026=ORIENTED_EDGE('',*,*,#7066,.T.);
#10027=ORIENTED_EDGE('',*,*,#7067,.T.);
#10028=ORIENTED_EDGE('',*,*,#7068,.F.);
#10029=ORIENTED_EDGE('',*,*,#7067,.F.);
#10030=ORIENTED_EDGE('',*,*,#7069,.T.);
#10031=ORIENTED_EDGE('',*,*,#7070,.T.);
#10032=ORIENTED_EDGE('',*,*,#7071,.F.);
#10033=ORIENTED_EDGE('',*,*,#7072,.F.);
#10034=ORIENTED_EDGE('',*,*,#7073,.T.);
#10035=ORIENTED_EDGE('',*,*,#7072,.T.);
#10036=ORIENTED_EDGE('',*,*,#7074,.F.);
#10037=ORIENTED_EDGE('',*,*,#7075,.F.);
#10038=ORIENTED_EDGE('',*,*,#7076,.T.);
#10039=ORIENTED_EDGE('',*,*,#7075,.T.);
#10040=ORIENTED_EDGE('',*,*,#7077,.F.);
#10041=ORIENTED_EDGE('',*,*,#7078,.F.);
#10042=ORIENTED_EDGE('',*,*,#7079,.T.);
#10043=ORIENTED_EDGE('',*,*,#7078,.T.);
#10044=ORIENTED_EDGE('',*,*,#7080,.F.);
#10045=ORIENTED_EDGE('',*,*,#7070,.F.);
#10046=ORIENTED_EDGE('',*,*,#7081,.T.);
#10047=ORIENTED_EDGE('',*,*,#7082,.T.);
#10048=ORIENTED_EDGE('',*,*,#7083,.F.);
#10049=ORIENTED_EDGE('',*,*,#7082,.F.);
#10050=ORIENTED_EDGE('',*,*,#7084,.T.);
#10051=ORIENTED_EDGE('',*,*,#7085,.T.);
#10052=ORIENTED_EDGE('',*,*,#7086,.F.);
#10053=ORIENTED_EDGE('',*,*,#7085,.F.);
#10054=ORIENTED_EDGE('',*,*,#7087,.T.);
#10055=ORIENTED_EDGE('',*,*,#7088,.T.);
#10056=ORIENTED_EDGE('',*,*,#7089,.F.);
#10057=ORIENTED_EDGE('',*,*,#7090,.F.);
#10058=ORIENTED_EDGE('',*,*,#7091,.T.);
#10059=ORIENTED_EDGE('',*,*,#7090,.T.);
#10060=ORIENTED_EDGE('',*,*,#7092,.F.);
#10061=ORIENTED_EDGE('',*,*,#7093,.F.);
#10062=ORIENTED_EDGE('',*,*,#7094,.T.);
#10063=ORIENTED_EDGE('',*,*,#7093,.T.);
#10064=ORIENTED_EDGE('',*,*,#7095,.F.);
#10065=ORIENTED_EDGE('',*,*,#7096,.F.);
#10066=ORIENTED_EDGE('',*,*,#7097,.T.);
#10067=ORIENTED_EDGE('',*,*,#7096,.T.);
#10068=ORIENTED_EDGE('',*,*,#7098,.F.);
#10069=ORIENTED_EDGE('',*,*,#7088,.F.);
#10070=ORIENTED_EDGE('',*,*,#7099,.T.);
#10071=ORIENTED_EDGE('',*,*,#7100,.T.);
#10072=ORIENTED_EDGE('',*,*,#7101,.F.);
#10073=ORIENTED_EDGE('',*,*,#7102,.F.);
#10074=ORIENTED_EDGE('',*,*,#7103,.T.);
#10075=ORIENTED_EDGE('',*,*,#7102,.T.);
#10076=ORIENTED_EDGE('',*,*,#7104,.F.);
#10077=ORIENTED_EDGE('',*,*,#7105,.F.);
#10078=ORIENTED_EDGE('',*,*,#7106,.T.);
#10079=ORIENTED_EDGE('',*,*,#7105,.T.);
#10080=ORIENTED_EDGE('',*,*,#7107,.F.);
#10081=ORIENTED_EDGE('',*,*,#7108,.F.);
#10082=ORIENTED_EDGE('',*,*,#7109,.T.);
#10083=ORIENTED_EDGE('',*,*,#7108,.T.);
#10084=ORIENTED_EDGE('',*,*,#7110,.F.);
#10085=ORIENTED_EDGE('',*,*,#7100,.F.);
#10086=ORIENTED_EDGE('',*,*,#7111,.T.);
#10087=ORIENTED_EDGE('',*,*,#7112,.T.);
#10088=ORIENTED_EDGE('',*,*,#7113,.F.);
#10089=ORIENTED_EDGE('',*,*,#7114,.F.);
#10090=ORIENTED_EDGE('',*,*,#7115,.T.);
#10091=ORIENTED_EDGE('',*,*,#7114,.T.);
#10092=ORIENTED_EDGE('',*,*,#7116,.F.);
#10093=ORIENTED_EDGE('',*,*,#7117,.F.);
#10094=ORIENTED_EDGE('',*,*,#7118,.T.);
#10095=ORIENTED_EDGE('',*,*,#7117,.T.);
#10096=ORIENTED_EDGE('',*,*,#7119,.F.);
#10097=ORIENTED_EDGE('',*,*,#7120,.F.);
#10098=ORIENTED_EDGE('',*,*,#7121,.T.);
#10099=ORIENTED_EDGE('',*,*,#7120,.T.);
#10100=ORIENTED_EDGE('',*,*,#7122,.F.);
#10101=ORIENTED_EDGE('',*,*,#7112,.F.);
#10102=ORIENTED_EDGE('',*,*,#7123,.T.);
#10103=ORIENTED_EDGE('',*,*,#7124,.T.);
#10104=ORIENTED_EDGE('',*,*,#7125,.F.);
#10105=ORIENTED_EDGE('',*,*,#7126,.F.);
#10106=ORIENTED_EDGE('',*,*,#7127,.T.);
#10107=ORIENTED_EDGE('',*,*,#7126,.T.);
#10108=ORIENTED_EDGE('',*,*,#7128,.F.);
#10109=ORIENTED_EDGE('',*,*,#7129,.F.);
#10110=ORIENTED_EDGE('',*,*,#7130,.T.);
#10111=ORIENTED_EDGE('',*,*,#7129,.T.);
#10112=ORIENTED_EDGE('',*,*,#7131,.F.);
#10113=ORIENTED_EDGE('',*,*,#7132,.F.);
#10114=ORIENTED_EDGE('',*,*,#7133,.T.);
#10115=ORIENTED_EDGE('',*,*,#7132,.T.);
#10116=ORIENTED_EDGE('',*,*,#7134,.F.);
#10117=ORIENTED_EDGE('',*,*,#7124,.F.);
#10118=ORIENTED_EDGE('',*,*,#7135,.T.);
#10119=ORIENTED_EDGE('',*,*,#7136,.T.);
#10120=ORIENTED_EDGE('',*,*,#7137,.F.);
#10121=ORIENTED_EDGE('',*,*,#7136,.F.);
#10122=ORIENTED_EDGE('',*,*,#7138,.T.);
#10123=ORIENTED_EDGE('',*,*,#7139,.T.);
#10124=ORIENTED_EDGE('',*,*,#7140,.F.);
#10125=ORIENTED_EDGE('',*,*,#7139,.F.);
#10126=ORIENTED_EDGE('',*,*,#7141,.F.);
#10127=ORIENTED_EDGE('',*,*,#7142,.T.);
#10128=ORIENTED_EDGE('',*,*,#7143,.F.);
#10129=ORIENTED_EDGE('',*,*,#7144,.F.);
#10130=ORIENTED_EDGE('',*,*,#7145,.T.);
#10131=ORIENTED_EDGE('',*,*,#7144,.T.);
#10132=ORIENTED_EDGE('',*,*,#7146,.F.);
#10133=ORIENTED_EDGE('',*,*,#7147,.F.);
#10134=ORIENTED_EDGE('',*,*,#7148,.F.);
#10135=ORIENTED_EDGE('',*,*,#7147,.T.);
#10136=ORIENTED_EDGE('',*,*,#7149,.F.);
#10137=ORIENTED_EDGE('',*,*,#7150,.F.);
#10138=ORIENTED_EDGE('',*,*,#7151,.T.);
#10139=ORIENTED_EDGE('',*,*,#7150,.T.);
#10140=ORIENTED_EDGE('',*,*,#7152,.F.);
#10141=ORIENTED_EDGE('',*,*,#7153,.F.);
#10142=ORIENTED_EDGE('',*,*,#7154,.F.);
#10143=ORIENTED_EDGE('',*,*,#7153,.T.);
#10144=ORIENTED_EDGE('',*,*,#7155,.F.);
#10145=ORIENTED_EDGE('',*,*,#7156,.F.);
#10146=ORIENTED_EDGE('',*,*,#7157,.T.);
#10147=ORIENTED_EDGE('',*,*,#7156,.T.);
#10148=ORIENTED_EDGE('',*,*,#7158,.F.);
#10149=ORIENTED_EDGE('',*,*,#7159,.F.);
#10150=ORIENTED_EDGE('',*,*,#7160,.F.);
#10151=ORIENTED_EDGE('',*,*,#7159,.T.);
#10152=ORIENTED_EDGE('',*,*,#7161,.F.);
#10153=ORIENTED_EDGE('',*,*,#7162,.F.);
#10154=ORIENTED_EDGE('',*,*,#7163,.T.);
#10155=ORIENTED_EDGE('',*,*,#7162,.T.);
#10156=ORIENTED_EDGE('',*,*,#7164,.F.);
#10157=ORIENTED_EDGE('',*,*,#7142,.F.);
#10158=ORIENTED_EDGE('',*,*,#7164,.T.);
#10159=ORIENTED_EDGE('',*,*,#7161,.T.);
#10160=ORIENTED_EDGE('',*,*,#7158,.T.);
#10161=ORIENTED_EDGE('',*,*,#7155,.T.);
#10162=ORIENTED_EDGE('',*,*,#7152,.T.);
#10163=ORIENTED_EDGE('',*,*,#7149,.T.);
#10164=ORIENTED_EDGE('',*,*,#7146,.T.);
#10165=ORIENTED_EDGE('',*,*,#7143,.T.);
#10166=ORIENTED_EDGE('',*,*,#7140,.T.);
#10167=ORIENTED_EDGE('',*,*,#7137,.T.);
#10168=ORIENTED_EDGE('',*,*,#7134,.T.);
#10169=ORIENTED_EDGE('',*,*,#7131,.T.);
#10170=ORIENTED_EDGE('',*,*,#7128,.T.);
#10171=ORIENTED_EDGE('',*,*,#7125,.T.);
#10172=ORIENTED_EDGE('',*,*,#7122,.T.);
#10173=ORIENTED_EDGE('',*,*,#7119,.T.);
#10174=ORIENTED_EDGE('',*,*,#7116,.T.);
#10175=ORIENTED_EDGE('',*,*,#7113,.T.);
#10176=ORIENTED_EDGE('',*,*,#7110,.T.);
#10177=ORIENTED_EDGE('',*,*,#7107,.T.);
#10178=ORIENTED_EDGE('',*,*,#7104,.T.);
#10179=ORIENTED_EDGE('',*,*,#7101,.T.);
#10180=ORIENTED_EDGE('',*,*,#7098,.T.);
#10181=ORIENTED_EDGE('',*,*,#7095,.T.);
#10182=ORIENTED_EDGE('',*,*,#7092,.T.);
#10183=ORIENTED_EDGE('',*,*,#7089,.T.);
#10184=ORIENTED_EDGE('',*,*,#7086,.T.);
#10185=ORIENTED_EDGE('',*,*,#7083,.T.);
#10186=ORIENTED_EDGE('',*,*,#7080,.T.);
#10187=ORIENTED_EDGE('',*,*,#7077,.T.);
#10188=ORIENTED_EDGE('',*,*,#7074,.T.);
#10189=ORIENTED_EDGE('',*,*,#7071,.T.);
#10190=ORIENTED_EDGE('',*,*,#7068,.T.);
#10191=ORIENTED_EDGE('',*,*,#7065,.T.);
#10192=ORIENTED_EDGE('',*,*,#7062,.T.);
#10193=ORIENTED_EDGE('',*,*,#7059,.T.);
#10194=ORIENTED_EDGE('',*,*,#7056,.T.);
#10195=ORIENTED_EDGE('',*,*,#7053,.T.);
#10196=ORIENTED_EDGE('',*,*,#7050,.T.);
#10197=ORIENTED_EDGE('',*,*,#7047,.T.);
#10198=ORIENTED_EDGE('',*,*,#7044,.T.);
#10199=ORIENTED_EDGE('',*,*,#7041,.T.);
#10200=ORIENTED_EDGE('',*,*,#7038,.T.);
#10201=ORIENTED_EDGE('',*,*,#7035,.T.);
#10202=ORIENTED_EDGE('',*,*,#7032,.T.);
#10203=ORIENTED_EDGE('',*,*,#7029,.T.);
#10204=ORIENTED_EDGE('',*,*,#7026,.T.);
#10205=ORIENTED_EDGE('',*,*,#7023,.T.);
#10206=ORIENTED_EDGE('',*,*,#7020,.T.);
#10207=ORIENTED_EDGE('',*,*,#7017,.T.);
#10208=ORIENTED_EDGE('',*,*,#7014,.T.);
#10209=ORIENTED_EDGE('',*,*,#7011,.T.);
#10210=ORIENTED_EDGE('',*,*,#7008,.T.);
#10211=ORIENTED_EDGE('',*,*,#7005,.T.);
#10212=ORIENTED_EDGE('',*,*,#7002,.T.);
#10213=ORIENTED_EDGE('',*,*,#7163,.F.);
#10214=ORIENTED_EDGE('',*,*,#7141,.T.);
#10215=ORIENTED_EDGE('',*,*,#7145,.F.);
#10216=ORIENTED_EDGE('',*,*,#7148,.T.);
#10217=ORIENTED_EDGE('',*,*,#7151,.F.);
#10218=ORIENTED_EDGE('',*,*,#7154,.T.);
#10219=ORIENTED_EDGE('',*,*,#7157,.F.);
#10220=ORIENTED_EDGE('',*,*,#7160,.T.);
#10221=ORIENTED_EDGE('',*,*,#7138,.F.);
#10222=ORIENTED_EDGE('',*,*,#7135,.F.);
#10223=ORIENTED_EDGE('',*,*,#7133,.F.);
#10224=ORIENTED_EDGE('',*,*,#7123,.F.);
#10225=ORIENTED_EDGE('',*,*,#7127,.F.);
#10226=ORIENTED_EDGE('',*,*,#7130,.F.);
#10227=ORIENTED_EDGE('',*,*,#7121,.F.);
#10228=ORIENTED_EDGE('',*,*,#7111,.F.);
#10229=ORIENTED_EDGE('',*,*,#7115,.F.);
#10230=ORIENTED_EDGE('',*,*,#7118,.F.);
#10231=ORIENTED_EDGE('',*,*,#7109,.F.);
#10232=ORIENTED_EDGE('',*,*,#7099,.F.);
#10233=ORIENTED_EDGE('',*,*,#7103,.F.);
#10234=ORIENTED_EDGE('',*,*,#7106,.F.);
#10235=ORIENTED_EDGE('',*,*,#7097,.F.);
#10236=ORIENTED_EDGE('',*,*,#7087,.F.);
#10237=ORIENTED_EDGE('',*,*,#7091,.F.);
#10238=ORIENTED_EDGE('',*,*,#7094,.F.);
#10239=ORIENTED_EDGE('',*,*,#7084,.F.);
#10240=ORIENTED_EDGE('',*,*,#7081,.F.);
#10241=ORIENTED_EDGE('',*,*,#7079,.F.);
#10242=ORIENTED_EDGE('',*,*,#7069,.F.);
#10243=ORIENTED_EDGE('',*,*,#7073,.F.);
#10244=ORIENTED_EDGE('',*,*,#7076,.F.);
#10245=ORIENTED_EDGE('',*,*,#7066,.F.);
#10246=ORIENTED_EDGE('',*,*,#7063,.F.);
#10247=ORIENTED_EDGE('',*,*,#7060,.F.);
#10248=ORIENTED_EDGE('',*,*,#7057,.F.);
#10249=ORIENTED_EDGE('',*,*,#7054,.F.);
#10250=ORIENTED_EDGE('',*,*,#7052,.F.);
#10251=ORIENTED_EDGE('',*,*,#7042,.F.);
#10252=ORIENTED_EDGE('',*,*,#7046,.F.);
#10253=ORIENTED_EDGE('',*,*,#7049,.F.);
#10254=ORIENTED_EDGE('',*,*,#7040,.F.);
#10255=ORIENTED_EDGE('',*,*,#7030,.F.);
#10256=ORIENTED_EDGE('',*,*,#7034,.F.);
#10257=ORIENTED_EDGE('',*,*,#7037,.F.);
#10258=ORIENTED_EDGE('',*,*,#7027,.F.);
#10259=ORIENTED_EDGE('',*,*,#7024,.F.);
#10260=ORIENTED_EDGE('',*,*,#7021,.F.);
#10261=ORIENTED_EDGE('',*,*,#7018,.F.);
#10262=ORIENTED_EDGE('',*,*,#7015,.F.);
#10263=ORIENTED_EDGE('',*,*,#7013,.F.);
#10264=ORIENTED_EDGE('',*,*,#7003,.F.);
#10265=ORIENTED_EDGE('',*,*,#7007,.F.);
#10266=ORIENTED_EDGE('',*,*,#7010,.F.);
#10267=ORIENTED_EDGE('',*,*,#7000,.F.);
#10603=CYLINDRICAL_SURFACE('',#12232,2.5);
#10604=CYLINDRICAL_SURFACE('',#12236,1.3925055570925);
#10605=CYLINDRICAL_SURFACE('',#12240,1.3925055570925);
#10606=CYLINDRICAL_SURFACE('',#12243,2.46675107308807);
#10607=CYLINDRICAL_SURFACE('',#12246,2.46675107308807);
#10608=CYLINDRICAL_SURFACE('',#12249,2.46675107308807);
#10609=CYLINDRICAL_SURFACE('',#12252,2.46675107308807);
#10610=CYLINDRICAL_SURFACE('',#12255,2.46675107308807);
#10611=CYLINDRICAL_SURFACE('',#12259,2.69990459756453);
#10612=CYLINDRICAL_SURFACE('',#12263,2.69990459756453);
#10613=CYLINDRICAL_SURFACE('',#12267,1.3925055570925);
#10614=CYLINDRICAL_SURFACE('',#12271,1.3925055570925);
#10615=CYLINDRICAL_SURFACE('',#12274,2.5);
#10616=CYLINDRICAL_SURFACE('',#12277,2.46675107308807);
#10617=CYLINDRICAL_SURFACE('',#12280,2.5);
#10618=CYLINDRICAL_SURFACE('',#12283,2.46675107308807);
#10619=CYLINDRICAL_SURFACE('',#12286,2.46675107308807);
#10620=CYLINDRICAL_SURFACE('',#12290,1.3925055570925);
#10621=CYLINDRICAL_SURFACE('',#12294,1.3925055570925);
#10622=CYLINDRICAL_SURFACE('',#12297,2.5);
#10623=CYLINDRICAL_SURFACE('',#12300,2.46675107308807);
#10624=CYLINDRICAL_SURFACE('',#12304,1.3925055570925);
#10625=CYLINDRICAL_SURFACE('',#12308,1.3925055570925);
#10626=CYLINDRICAL_SURFACE('',#12312,1.3925055570925);
#10627=CYLINDRICAL_SURFACE('',#12316,1.3925055570925);
#10628=CYLINDRICAL_SURFACE('',#12320,1.3925055570925);
#10629=CYLINDRICAL_SURFACE('',#12324,1.3925055570925);
#10630=CYLINDRICAL_SURFACE('',#12328,2.69990459756453);
#10631=CYLINDRICAL_SURFACE('',#12332,2.69990459756453);
#10632=CYLINDRICAL_SURFACE('',#12335,2.46675107308807);
#10633=CYLINDRICAL_SURFACE('',#12338,2.46675107308807);
#10634=CYLINDRICAL_SURFACE('',#12342,3.00000000000004);
#10635=CYLINDRICAL_SURFACE('',#12346,3.00000000000003);
#10636=CYLINDRICAL_SURFACE('',#12350,3.00000000000004);
#10637=CYLINDRICAL_SURFACE('',#12354,3.00000000000004);
#11171=ADVANCED_FACE('',(#1550),#10603,.F.);
#11172=ADVANCED_FACE('',(#1551),#671,.T.);
#11173=ADVANCED_FACE('',(#1552),#10604,.F.);
#11174=ADVANCED_FACE('',(#1553),#672,.T.);
#11175=ADVANCED_FACE('',(#1554),#10605,.F.);
#11176=ADVANCED_FACE('',(#1555),#10606,.F.);
#11177=ADVANCED_FACE('',(#1556),#10607,.F.);
#11178=ADVANCED_FACE('',(#1557),#10608,.F.);
#11179=ADVANCED_FACE('',(#1558),#10609,.F.);
#11180=ADVANCED_FACE('',(#1559),#10610,.F.);
#11181=ADVANCED_FACE('',(#1560),#673,.T.);
#11182=ADVANCED_FACE('',(#1561),#10611,.F.);
#11183=ADVANCED_FACE('',(#1562),#674,.T.);
#11184=ADVANCED_FACE('',(#1563),#10612,.F.);
#11185=ADVANCED_FACE('',(#1564),#675,.T.);
#11186=ADVANCED_FACE('',(#1565),#10613,.F.);
#11187=ADVANCED_FACE('',(#1566),#676,.T.);
#11188=ADVANCED_FACE('',(#1567),#10614,.F.);
#11189=ADVANCED_FACE('',(#1568),#10615,.F.);
#11190=ADVANCED_FACE('',(#1569),#10616,.F.);
#11191=ADVANCED_FACE('',(#1570),#10617,.F.);
#11192=ADVANCED_FACE('',(#1571),#10618,.F.);
#11193=ADVANCED_FACE('',(#1572),#10619,.F.);
#11194=ADVANCED_FACE('',(#1573),#677,.T.);
#11195=ADVANCED_FACE('',(#1574),#10620,.F.);
#11196=ADVANCED_FACE('',(#1575),#678,.T.);
#11197=ADVANCED_FACE('',(#1576),#10621,.F.);
#11198=ADVANCED_FACE('',(#1577),#10622,.F.);
#11199=ADVANCED_FACE('',(#1578),#10623,.F.);
#11200=ADVANCED_FACE('',(#1579),#679,.T.);
#11201=ADVANCED_FACE('',(#1580),#10624,.F.);
#11202=ADVANCED_FACE('',(#1581),#680,.T.);
#11203=ADVANCED_FACE('',(#1582),#10625,.F.);
#11204=ADVANCED_FACE('',(#1583),#681,.T.);
#11205=ADVANCED_FACE('',(#1584),#10626,.F.);
#11206=ADVANCED_FACE('',(#1585),#682,.T.);
#11207=ADVANCED_FACE('',(#1586),#10627,.F.);
#11208=ADVANCED_FACE('',(#1587),#683,.T.);
#11209=ADVANCED_FACE('',(#1588),#10628,.F.);
#11210=ADVANCED_FACE('',(#1589),#684,.T.);
#11211=ADVANCED_FACE('',(#1590),#10629,.F.);
#11212=ADVANCED_FACE('',(#1591),#685,.T.);
#11213=ADVANCED_FACE('',(#1592),#10630,.F.);
#11214=ADVANCED_FACE('',(#1593),#686,.T.);
#11215=ADVANCED_FACE('',(#1594),#10631,.F.);
#11216=ADVANCED_FACE('',(#1595),#10632,.F.);
#11217=ADVANCED_FACE('',(#1596),#10633,.F.);
#11218=ADVANCED_FACE('',(#1597),#687,.T.);
#11219=ADVANCED_FACE('',(#1598),#10634,.T.);
#11220=ADVANCED_FACE('',(#1599),#688,.T.);
#11221=ADVANCED_FACE('',(#1600),#10635,.T.);
#11222=ADVANCED_FACE('',(#1601),#689,.T.);
#11223=ADVANCED_FACE('',(#1602),#10636,.T.);
#11224=ADVANCED_FACE('',(#1603),#690,.T.);
#11225=ADVANCED_FACE('',(#1604),#10637,.T.);
#11226=ADVANCED_FACE('',(#1605,#207,#208,#209,#210,#211,#212,#213,#214,
#215,#216,#217,#218,#219,#220,#221,#222,#223,#224,#225,#226,#227,#228,#229),
#691,.T.);
#11227=ADVANCED_FACE('',(#1606,#230,#231,#232,#233,#234,#235,#236,#237,
#238,#239,#240,#241,#242,#243,#244,#245,#246,#247,#248,#249,#250,#251,#252),
#692,.F.);
#11291=CLOSED_SHELL('',(#11171,#11172,#11173,#11174,#11175,#11176,#11177,
#11178,#11179,#11180,#11181,#11182,#11183,#11184,#11185,#11186,#11187,#11188,
#11189,#11190,#11191,#11192,#11193,#11194,#11195,#11196,#11197,#11198,#11199,
#11200,#11201,#11202,#11203,#11204,#11205,#11206,#11207,#11208,#11209,#11210,
#11211,#11212,#11213,#11214,#11215,#11216,#11217,#11218,#11219,#11220,#11221,
#11222,#11223,#11224,#11225,#11226,#11227));
#12231=AXIS2_PLACEMENT_3D('',#35926,#14827,#14828);
#12232=AXIS2_PLACEMENT_3D('',#35927,#14829,#14830);
#12233=AXIS2_PLACEMENT_3D('',#35929,#14831,#14832);
#12234=AXIS2_PLACEMENT_3D('',#35932,#14834,#14835);
#12235=AXIS2_PLACEMENT_3D('',#35933,#14836,#14837);
#12236=AXIS2_PLACEMENT_3D('',#35942,#14842,#14843);
#12237=AXIS2_PLACEMENT_3D('',#35944,#14844,#14845);
#12238=AXIS2_PLACEMENT_3D('',#35946,#14846,#14847);
#12239=AXIS2_PLACEMENT_3D('',#35948,#14849,#14850);
#12240=AXIS2_PLACEMENT_3D('',#35954,#14854,#14855);
#12241=AXIS2_PLACEMENT_3D('',#35955,#14856,#14857);
#12242=AXIS2_PLACEMENT_3D('',#35956,#14858,#14859);
#12243=AXIS2_PLACEMENT_3D('',#35957,#14860,#14861);
#12244=AXIS2_PLACEMENT_3D('',#35959,#14862,#14863);
#12245=AXIS2_PLACEMENT_3D('',#35962,#14865,#14866);
#12246=AXIS2_PLACEMENT_3D('',#35963,#14867,#14868);
#12247=AXIS2_PLACEMENT_3D('',#35965,#14869,#14870);
#12248=AXIS2_PLACEMENT_3D('',#35968,#14872,#14873);
#12249=AXIS2_PLACEMENT_3D('',#35969,#14874,#14875);
#12250=AXIS2_PLACEMENT_3D('',#35971,#14876,#14877);
#12251=AXIS2_PLACEMENT_3D('',#35974,#14879,#14880);
#12252=AXIS2_PLACEMENT_3D('',#35975,#14881,#14882);
#12253=AXIS2_PLACEMENT_3D('',#35977,#14883,#14884);
#12254=AXIS2_PLACEMENT_3D('',#35980,#14886,#14887);
#12255=AXIS2_PLACEMENT_3D('',#35981,#14888,#14889);
#12256=AXIS2_PLACEMENT_3D('',#35983,#14890,#14891);
#12257=AXIS2_PLACEMENT_3D('',#35986,#14893,#14894);
#12258=AXIS2_PLACEMENT_3D('',#35987,#14895,#14896);
#12259=AXIS2_PLACEMENT_3D('',#35996,#14901,#14902);
#12260=AXIS2_PLACEMENT_3D('',#35998,#14903,#14904);
#12261=AXIS2_PLACEMENT_3D('',#36000,#14905,#14906);
#12262=AXIS2_PLACEMENT_3D('',#36002,#14908,#14909);
#12263=AXIS2_PLACEMENT_3D('',#36008,#14913,#14914);
#12264=AXIS2_PLACEMENT_3D('',#36009,#14915,#14916);
#12265=AXIS2_PLACEMENT_3D('',#36010,#14917,#14918);
#12266=AXIS2_PLACEMENT_3D('',#36011,#14919,#14920);
#12267=AXIS2_PLACEMENT_3D('',#36020,#14925,#14926);
#12268=AXIS2_PLACEMENT_3D('',#36022,#14927,#14928);
#12269=AXIS2_PLACEMENT_3D('',#36024,#14929,#14930);
#12270=AXIS2_PLACEMENT_3D('',#36026,#14932,#14933);
#12271=AXIS2_PLACEMENT_3D('',#36032,#14937,#14938);
#12272=AXIS2_PLACEMENT_3D('',#36033,#14939,#14940);
#12273=AXIS2_PLACEMENT_3D('',#36034,#14941,#14942);
#12274=AXIS2_PLACEMENT_3D('',#36035,#14943,#14944);
#12275=AXIS2_PLACEMENT_3D('',#36037,#14945,#14946);
#12276=AXIS2_PLACEMENT_3D('',#36040,#14948,#14949);
#12277=AXIS2_PLACEMENT_3D('',#36041,#14950,#14951);
#12278=AXIS2_PLACEMENT_3D('',#36043,#14952,#14953);
#12279=AXIS2_PLACEMENT_3D('',#36046,#14955,#14956);
#12280=AXIS2_PLACEMENT_3D('',#36047,#14957,#14958);
#12281=AXIS2_PLACEMENT_3D('',#36049,#14959,#14960);
#12282=AXIS2_PLACEMENT_3D('',#36052,#14962,#14963);
#12283=AXIS2_PLACEMENT_3D('',#36053,#14964,#14965);
#12284=AXIS2_PLACEMENT_3D('',#36055,#14966,#14967);
#12285=AXIS2_PLACEMENT_3D('',#36058,#14969,#14970);
#12286=AXIS2_PLACEMENT_3D('',#36059,#14971,#14972);
#12287=AXIS2_PLACEMENT_3D('',#36061,#14973,#14974);
#12288=AXIS2_PLACEMENT_3D('',#36064,#14976,#14977);
#12289=AXIS2_PLACEMENT_3D('',#36065,#14978,#14979);
#12290=AXIS2_PLACEMENT_3D('',#36074,#14984,#14985);
#12291=AXIS2_PLACEMENT_3D('',#36076,#14986,#14987);
#12292=AXIS2_PLACEMENT_3D('',#36078,#14988,#14989);
#12293=AXIS2_PLACEMENT_3D('',#36080,#14991,#14992);
#12294=AXIS2_PLACEMENT_3D('',#36086,#14996,#14997);
#12295=AXIS2_PLACEMENT_3D('',#36087,#14998,#14999);
#12296=AXIS2_PLACEMENT_3D('',#36088,#15000,#15001);
#12297=AXIS2_PLACEMENT_3D('',#36089,#15002,#15003);
#12298=AXIS2_PLACEMENT_3D('',#36091,#15004,#15005);
#12299=AXIS2_PLACEMENT_3D('',#36094,#15007,#15008);
#12300=AXIS2_PLACEMENT_3D('',#36095,#15009,#15010);
#12301=AXIS2_PLACEMENT_3D('',#36097,#15011,#15012);
#12302=AXIS2_PLACEMENT_3D('',#36100,#15014,#15015);
#12303=AXIS2_PLACEMENT_3D('',#36101,#15016,#15017);
#12304=AXIS2_PLACEMENT_3D('',#36110,#15022,#15023);
#12305=AXIS2_PLACEMENT_3D('',#36112,#15024,#15025);
#12306=AXIS2_PLACEMENT_3D('',#36114,#15026,#15027);
#12307=AXIS2_PLACEMENT_3D('',#36116,#15029,#15030);
#12308=AXIS2_PLACEMENT_3D('',#36122,#15034,#15035);
#12309=AXIS2_PLACEMENT_3D('',#36123,#15036,#15037);
#12310=AXIS2_PLACEMENT_3D('',#36124,#15038,#15039);
#12311=AXIS2_PLACEMENT_3D('',#36125,#15040,#15041);
#12312=AXIS2_PLACEMENT_3D('',#36134,#15046,#15047);
#12313=AXIS2_PLACEMENT_3D('',#36136,#15048,#15049);
#12314=AXIS2_PLACEMENT_3D('',#36138,#15050,#15051);
#12315=AXIS2_PLACEMENT_3D('',#36140,#15053,#15054);
#12316=AXIS2_PLACEMENT_3D('',#36146,#15058,#15059);
#12317=AXIS2_PLACEMENT_3D('',#36147,#15060,#15061);
#12318=AXIS2_PLACEMENT_3D('',#36148,#15062,#15063);
#12319=AXIS2_PLACEMENT_3D('',#36149,#15064,#15065);
#12320=AXIS2_PLACEMENT_3D('',#36158,#15070,#15071);
#12321=AXIS2_PLACEMENT_3D('',#36160,#15072,#15073);
#12322=AXIS2_PLACEMENT_3D('',#36162,#15074,#15075);
#12323=AXIS2_PLACEMENT_3D('',#36164,#15077,#15078);
#12324=AXIS2_PLACEMENT_3D('',#36170,#15082,#15083);
#12325=AXIS2_PLACEMENT_3D('',#36171,#15084,#15085);
#12326=AXIS2_PLACEMENT_3D('',#36172,#15086,#15087);
#12327=AXIS2_PLACEMENT_3D('',#36173,#15088,#15089);
#12328=AXIS2_PLACEMENT_3D('',#36182,#15094,#15095);
#12329=AXIS2_PLACEMENT_3D('',#36184,#15096,#15097);
#12330=AXIS2_PLACEMENT_3D('',#36186,#15098,#15099);
#12331=AXIS2_PLACEMENT_3D('',#36188,#15101,#15102);
#12332=AXIS2_PLACEMENT_3D('',#36194,#15106,#15107);
#12333=AXIS2_PLACEMENT_3D('',#36195,#15108,#15109);
#12334=AXIS2_PLACEMENT_3D('',#36196,#15110,#15111);
#12335=AXIS2_PLACEMENT_3D('',#36197,#15112,#15113);
#12336=AXIS2_PLACEMENT_3D('',#36199,#15114,#15115);
#12337=AXIS2_PLACEMENT_3D('',#36202,#15117,#15118);
#12338=AXIS2_PLACEMENT_3D('',#36203,#15119,#15120);
#12339=AXIS2_PLACEMENT_3D('',#36205,#15121,#15122);
#12340=AXIS2_PLACEMENT_3D('',#36208,#15124,#15125);
#12341=AXIS2_PLACEMENT_3D('',#36209,#15126,#15127);
#12342=AXIS2_PLACEMENT_3D('',#36218,#15132,#15133);
#12343=AXIS2_PLACEMENT_3D('',#36220,#15134,#15135);
#12344=AXIS2_PLACEMENT_3D('',#36222,#15136,#15137);
#12345=AXIS2_PLACEMENT_3D('',#36224,#15139,#15140);
#12346=AXIS2_PLACEMENT_3D('',#36230,#15144,#15145);
#12347=AXIS2_PLACEMENT_3D('',#36232,#15146,#15147);
#12348=AXIS2_PLACEMENT_3D('',#36234,#15148,#15149);
#12349=AXIS2_PLACEMENT_3D('',#36236,#15151,#15152);
#12350=AXIS2_PLACEMENT_3D('',#36242,#15156,#15157);
#12351=AXIS2_PLACEMENT_3D('',#36244,#15158,#15159);
#12352=AXIS2_PLACEMENT_3D('',#36246,#15160,#15161);
#12353=AXIS2_PLACEMENT_3D('',#36248,#15163,#15164);
#12354=AXIS2_PLACEMENT_3D('',#36254,#15168,#15169);
#12355=AXIS2_PLACEMENT_3D('',#36255,#15170,#15171);
#12356=AXIS2_PLACEMENT_3D('',#36256,#15172,#15173);
#12357=AXIS2_PLACEMENT_3D('',#36257,#15174,#15175);
#12358=AXIS2_PLACEMENT_3D('',#36258,#15176,#15177);
#14827=DIRECTION('axis',(0.,0.,1.));
#14828=DIRECTION('refdir',(1.,0.,0.));
#14829=DIRECTION('center_axis',(-1.,0.,0.));
#14830=DIRECTION('ref_axis',(0.,-1.,0.));
#14831=DIRECTION('center_axis',(1.,0.,0.));
#14832=DIRECTION('ref_axis',(0.,-1.,0.));
#14833=DIRECTION('',(-1.,0.,0.));
#14834=DIRECTION('center_axis',(1.,0.,0.));
#14835=DIRECTION('ref_axis',(0.,-1.,0.));
#14836=DIRECTION('center_axis',(0.,1.,0.));
#14837=DIRECTION('ref_axis',(0.,0.,-1.));
#14838=DIRECTION('',(0.,0.,-1.));
#14839=DIRECTION('',(-1.,0.,0.));
#14840=DIRECTION('',(0.,0.,-1.));
#14841=DIRECTION('',(-1.,0.,0.));
#14842=DIRECTION('center_axis',(-1.,0.,0.));
#14843=DIRECTION('ref_axis',(0.,-1.,0.));
#14844=DIRECTION('center_axis',(1.,0.,0.));
#14845=DIRECTION('ref_axis',(0.,-1.,0.));
#14846=DIRECTION('center_axis',(1.,0.,0.));
#14847=DIRECTION('ref_axis',(0.,-1.,0.));
#14848=DIRECTION('',(-1.,0.,0.));
#14849=DIRECTION('center_axis',(0.,-1.,0.));
#14850=DIRECTION('ref_axis',(0.,0.,1.));
#14851=DIRECTION('',(0.,0.,1.));
#14852=DIRECTION('',(0.,0.,1.));
#14853=DIRECTION('',(-1.,0.,0.));
#14854=DIRECTION('center_axis',(-1.,0.,0.));
#14855=DIRECTION('ref_axis',(0.,1.,0.));
#14856=DIRECTION('center_axis',(1.,0.,0.));
#14857=DIRECTION('ref_axis',(0.,1.,0.));
#14858=DIRECTION('center_axis',(1.,0.,0.));
#14859=DIRECTION('ref_axis',(0.,1.,0.));
#14860=DIRECTION('center_axis',(-1.,0.,0.));
#14861=DIRECTION('ref_axis',(0.,-1.,0.));
#14862=DIRECTION('center_axis',(1.,0.,0.));
#14863=DIRECTION('ref_axis',(0.,-1.,0.));
#14864=DIRECTION('',(-1.,0.,0.));
#14865=DIRECTION('center_axis',(1.,0.,0.));
#14866=DIRECTION('ref_axis',(0.,-1.,0.));
#14867=DIRECTION('center_axis',(-1.,0.,0.));
#14868=DIRECTION('ref_axis',(0.,-1.,0.));
#14869=DIRECTION('center_axis',(1.,0.,0.));
#14870=DIRECTION('ref_axis',(0.,-1.,0.));
#14871=DIRECTION('',(-1.,0.,0.));
#14872=DIRECTION('center_axis',(1.,0.,0.));
#14873=DIRECTION('ref_axis',(0.,-1.,0.));
#14874=DIRECTION('center_axis',(-1.,0.,0.));
#14875=DIRECTION('ref_axis',(0.,-1.,0.));
#14876=DIRECTION('center_axis',(1.,0.,0.));
#14877=DIRECTION('ref_axis',(0.,-1.,0.));
#14878=DIRECTION('',(-1.,0.,0.));
#14879=DIRECTION('center_axis',(1.,0.,0.));
#14880=DIRECTION('ref_axis',(0.,-1.,0.));
#14881=DIRECTION('center_axis',(-1.,0.,0.));
#14882=DIRECTION('ref_axis',(0.,-1.,0.));
#14883=DIRECTION('center_axis',(1.,0.,0.));
#14884=DIRECTION('ref_axis',(0.,-1.,0.));
#14885=DIRECTION('',(-1.,0.,0.));
#14886=DIRECTION('center_axis',(1.,0.,0.));
#14887=DIRECTION('ref_axis',(0.,-1.,0.));
#14888=DIRECTION('center_axis',(-1.,0.,0.));
#14889=DIRECTION('ref_axis',(0.,-1.,0.));
#14890=DIRECTION('center_axis',(1.,0.,0.));
#14891=DIRECTION('ref_axis',(0.,-1.,0.));
#14892=DIRECTION('',(-1.,0.,0.));
#14893=DIRECTION('center_axis',(1.,0.,0.));
#14894=DIRECTION('ref_axis',(0.,-1.,0.));
#14895=DIRECTION('center_axis',(0.,1.,0.));
#14896=DIRECTION('ref_axis',(0.,0.,-1.));
#14897=DIRECTION('',(0.,0.,-1.));
#14898=DIRECTION('',(-1.,0.,0.));
#14899=DIRECTION('',(0.,0.,-1.));
#14900=DIRECTION('',(-1.,0.,0.));
#14901=DIRECTION('center_axis',(-1.,0.,0.));
#14902=DIRECTION('ref_axis',(0.,-1.,0.));
#14903=DIRECTION('center_axis',(1.,0.,0.));
#14904=DIRECTION('ref_axis',(0.,-1.,0.));
#14905=DIRECTION('center_axis',(1.,0.,0.));
#14906=DIRECTION('ref_axis',(0.,-1.,0.));
#14907=DIRECTION('',(-1.,0.,0.));
#14908=DIRECTION('center_axis',(0.,-1.,0.));
#14909=DIRECTION('ref_axis',(0.,0.,1.));
#14910=DIRECTION('',(0.,0.,1.));
#14911=DIRECTION('',(0.,0.,1.));
#14912=DIRECTION('',(-1.,0.,0.));
#14913=DIRECTION('center_axis',(-1.,0.,0.));
#14914=DIRECTION('ref_axis',(0.,1.,0.));
#14915=DIRECTION('center_axis',(1.,0.,0.));
#14916=DIRECTION('ref_axis',(0.,1.,0.));
#14917=DIRECTION('center_axis',(1.,0.,0.));
#14918=DIRECTION('ref_axis',(0.,1.,0.));
#14919=DIRECTION('center_axis',(0.,1.,0.));
#14920=DIRECTION('ref_axis',(0.,0.,-1.));
#14921=DIRECTION('',(0.,0.,-1.));
#14922=DIRECTION('',(-1.,0.,0.));
#14923=DIRECTION('',(0.,0.,-1.));
#14924=DIRECTION('',(-1.,0.,0.));
#14925=DIRECTION('center_axis',(-1.,0.,0.));
#14926=DIRECTION('ref_axis',(0.,-1.,0.));
#14927=DIRECTION('center_axis',(1.,0.,0.));
#14928=DIRECTION('ref_axis',(0.,-1.,0.));
#14929=DIRECTION('center_axis',(1.,0.,0.));
#14930=DIRECTION('ref_axis',(0.,-1.,0.));
#14931=DIRECTION('',(-1.,0.,0.));
#14932=DIRECTION('center_axis',(0.,-1.,0.));
#14933=DIRECTION('ref_axis',(0.,0.,1.));
#14934=DIRECTION('',(0.,0.,1.));
#14935=DIRECTION('',(0.,0.,1.));
#14936=DIRECTION('',(-1.,0.,0.));
#14937=DIRECTION('center_axis',(-1.,0.,0.));
#14938=DIRECTION('ref_axis',(0.,1.,0.));
#14939=DIRECTION('center_axis',(1.,0.,0.));
#14940=DIRECTION('ref_axis',(0.,1.,0.));
#14941=DIRECTION('center_axis',(1.,0.,0.));
#14942=DIRECTION('ref_axis',(0.,1.,0.));
#14943=DIRECTION('center_axis',(-1.,0.,0.));
#14944=DIRECTION('ref_axis',(0.,-1.,0.));
#14945=DIRECTION('center_axis',(1.,0.,0.));
#14946=DIRECTION('ref_axis',(0.,-1.,0.));
#14947=DIRECTION('',(-1.,0.,0.));
#14948=DIRECTION('center_axis',(1.,0.,0.));
#14949=DIRECTION('ref_axis',(0.,-1.,0.));
#14950=DIRECTION('center_axis',(-1.,0.,0.));
#14951=DIRECTION('ref_axis',(0.,-1.,0.));
#14952=DIRECTION('center_axis',(1.,0.,0.));
#14953=DIRECTION('ref_axis',(0.,-1.,0.));
#14954=DIRECTION('',(-1.,0.,0.));
#14955=DIRECTION('center_axis',(1.,0.,0.));
#14956=DIRECTION('ref_axis',(0.,-1.,0.));
#14957=DIRECTION('center_axis',(-1.,0.,0.));
#14958=DIRECTION('ref_axis',(0.,-1.,0.));
#14959=DIRECTION('center_axis',(1.,0.,0.));
#14960=DIRECTION('ref_axis',(0.,-1.,0.));
#14961=DIRECTION('',(-1.,0.,0.));
#14962=DIRECTION('center_axis',(1.,0.,0.));
#14963=DIRECTION('ref_axis',(0.,-1.,0.));
#14964=DIRECTION('center_axis',(-1.,0.,0.));
#14965=DIRECTION('ref_axis',(0.,-1.,0.));
#14966=DIRECTION('center_axis',(1.,0.,0.));
#14967=DIRECTION('ref_axis',(0.,-1.,0.));
#14968=DIRECTION('',(-1.,0.,0.));
#14969=DIRECTION('center_axis',(1.,0.,0.));
#14970=DIRECTION('ref_axis',(0.,-1.,0.));
#14971=DIRECTION('center_axis',(-1.,0.,0.));
#14972=DIRECTION('ref_axis',(0.,-1.,0.));
#14973=DIRECTION('center_axis',(1.,0.,0.));
#14974=DIRECTION('ref_axis',(0.,-1.,0.));
#14975=DIRECTION('',(-1.,0.,0.));
#14976=DIRECTION('center_axis',(1.,0.,0.));
#14977=DIRECTION('ref_axis',(0.,-1.,0.));
#14978=DIRECTION('center_axis',(0.,-1.,0.));
#14979=DIRECTION('ref_axis',(0.,0.,1.));
#14980=DIRECTION('',(0.,0.,1.));
#14981=DIRECTION('',(-1.,0.,0.));
#14982=DIRECTION('',(0.,0.,1.));
#14983=DIRECTION('',(-1.,0.,0.));
#14984=DIRECTION('center_axis',(-1.,0.,0.));
#14985=DIRECTION('ref_axis',(0.,1.,0.));
#14986=DIRECTION('center_axis',(1.,0.,0.));
#14987=DIRECTION('ref_axis',(0.,1.,0.));
#14988=DIRECTION('center_axis',(1.,0.,0.));
#14989=DIRECTION('ref_axis',(0.,1.,0.));
#14990=DIRECTION('',(-1.,0.,0.));
#14991=DIRECTION('center_axis',(0.,1.,0.));
#14992=DIRECTION('ref_axis',(0.,0.,-1.));
#14993=DIRECTION('',(0.,0.,-1.));
#14994=DIRECTION('',(0.,0.,-1.));
#14995=DIRECTION('',(-1.,0.,0.));
#14996=DIRECTION('center_axis',(-1.,0.,0.));
#14997=DIRECTION('ref_axis',(0.,-1.,0.));
#14998=DIRECTION('center_axis',(1.,0.,0.));
#14999=DIRECTION('ref_axis',(0.,-1.,0.));
#15000=DIRECTION('center_axis',(1.,0.,0.));
#15001=DIRECTION('ref_axis',(0.,-1.,0.));
#15002=DIRECTION('center_axis',(-1.,0.,0.));
#15003=DIRECTION('ref_axis',(0.,-1.,0.));
#15004=DIRECTION('center_axis',(1.,0.,0.));
#15005=DIRECTION('ref_axis',(0.,-1.,0.));
#15006=DIRECTION('',(-1.,0.,0.));
#15007=DIRECTION('center_axis',(1.,0.,0.));
#15008=DIRECTION('ref_axis',(0.,-1.,0.));
#15009=DIRECTION('center_axis',(-1.,0.,0.));
#15010=DIRECTION('ref_axis',(0.,-1.,0.));
#15011=DIRECTION('center_axis',(1.,0.,0.));
#15012=DIRECTION('ref_axis',(0.,-1.,0.));
#15013=DIRECTION('',(-1.,0.,0.));
#15014=DIRECTION('center_axis',(1.,0.,0.));
#15015=DIRECTION('ref_axis',(0.,-1.,0.));
#15016=DIRECTION('center_axis',(0.,1.,0.));
#15017=DIRECTION('ref_axis',(0.,0.,-1.));
#15018=DIRECTION('',(0.,0.,-1.));
#15019=DIRECTION('',(-1.,0.,0.));
#15020=DIRECTION('',(0.,0.,-1.));
#15021=DIRECTION('',(-1.,0.,0.));
#15022=DIRECTION('center_axis',(-1.,0.,0.));
#15023=DIRECTION('ref_axis',(0.,-1.,0.));
#15024=DIRECTION('center_axis',(1.,0.,0.));
#15025=DIRECTION('ref_axis',(0.,-1.,0.));
#15026=DIRECTION('center_axis',(1.,0.,0.));
#15027=DIRECTION('ref_axis',(0.,-1.,0.));
#15028=DIRECTION('',(-1.,0.,0.));
#15029=DIRECTION('center_axis',(0.,-1.,0.));
#15030=DIRECTION('ref_axis',(0.,0.,1.));
#15031=DIRECTION('',(0.,0.,1.));
#15032=DIRECTION('',(0.,0.,1.));
#15033=DIRECTION('',(-1.,0.,0.));
#15034=DIRECTION('center_axis',(-1.,0.,0.));
#15035=DIRECTION('ref_axis',(0.,1.,0.));
#15036=DIRECTION('center_axis',(1.,0.,0.));
#15037=DIRECTION('ref_axis',(0.,1.,0.));
#15038=DIRECTION('center_axis',(1.,0.,0.));
#15039=DIRECTION('ref_axis',(0.,1.,0.));
#15040=DIRECTION('center_axis',(0.,-1.,0.));
#15041=DIRECTION('ref_axis',(0.,0.,1.));
#15042=DIRECTION('',(0.,0.,1.));
#15043=DIRECTION('',(-1.,0.,0.));
#15044=DIRECTION('',(0.,0.,1.));
#15045=DIRECTION('',(-1.,0.,0.));
#15046=DIRECTION('center_axis',(-1.,0.,0.));
#15047=DIRECTION('ref_axis',(0.,1.,0.));
#15048=DIRECTION('center_axis',(1.,0.,0.));
#15049=DIRECTION('ref_axis',(0.,1.,0.));
#15050=DIRECTION('center_axis',(1.,0.,0.));
#15051=DIRECTION('ref_axis',(0.,1.,0.));
#15052=DIRECTION('',(-1.,0.,0.));
#15053=DIRECTION('center_axis',(0.,1.,0.));
#15054=DIRECTION('ref_axis',(0.,0.,-1.));
#15055=DIRECTION('',(0.,0.,-1.));
#15056=DIRECTION('',(0.,0.,-1.));
#15057=DIRECTION('',(-1.,0.,0.));
#15058=DIRECTION('center_axis',(-1.,0.,0.));
#15059=DIRECTION('ref_axis',(0.,-1.,0.));
#15060=DIRECTION('center_axis',(1.,0.,0.));
#15061=DIRECTION('ref_axis',(0.,-1.,0.));
#15062=DIRECTION('center_axis',(1.,0.,0.));
#15063=DIRECTION('ref_axis',(0.,-1.,0.));
#15064=DIRECTION('center_axis',(0.,1.,0.));
#15065=DIRECTION('ref_axis',(0.,0.,-1.));
#15066=DIRECTION('',(0.,0.,-1.));
#15067=DIRECTION('',(-1.,0.,0.));
#15068=DIRECTION('',(0.,0.,-1.));
#15069=DIRECTION('',(-1.,0.,0.));
#15070=DIRECTION('center_axis',(-1.,0.,0.));
#15071=DIRECTION('ref_axis',(0.,-1.,0.));
#15072=DIRECTION('center_axis',(1.,0.,0.));
#15073=DIRECTION('ref_axis',(0.,-1.,0.));
#15074=DIRECTION('center_axis',(1.,0.,0.));
#15075=DIRECTION('ref_axis',(0.,-1.,0.));
#15076=DIRECTION('',(-1.,0.,0.));
#15077=DIRECTION('center_axis',(0.,-1.,0.));
#15078=DIRECTION('ref_axis',(0.,0.,1.));
#15079=DIRECTION('',(0.,0.,1.));
#15080=DIRECTION('',(0.,0.,1.));
#15081=DIRECTION('',(-1.,0.,0.));
#15082=DIRECTION('center_axis',(-1.,0.,0.));
#15083=DIRECTION('ref_axis',(0.,1.,0.));
#15084=DIRECTION('center_axis',(1.,0.,0.));
#15085=DIRECTION('ref_axis',(0.,1.,0.));
#15086=DIRECTION('center_axis',(1.,0.,0.));
#15087=DIRECTION('ref_axis',(0.,1.,0.));
#15088=DIRECTION('center_axis',(0.,1.,0.));
#15089=DIRECTION('ref_axis',(0.,0.,-1.));
#15090=DIRECTION('',(0.,0.,-1.));
#15091=DIRECTION('',(-1.,0.,0.));
#15092=DIRECTION('',(0.,0.,-1.));
#15093=DIRECTION('',(-1.,0.,0.));
#15094=DIRECTION('center_axis',(-1.,0.,0.));
#15095=DIRECTION('ref_axis',(0.,-1.,0.));
#15096=DIRECTION('center_axis',(1.,0.,0.));
#15097=DIRECTION('ref_axis',(0.,-1.,0.));
#15098=DIRECTION('center_axis',(1.,0.,0.));
#15099=DIRECTION('ref_axis',(0.,-1.,0.));
#15100=DIRECTION('',(-1.,0.,0.));
#15101=DIRECTION('center_axis',(0.,-1.,0.));
#15102=DIRECTION('ref_axis',(0.,0.,1.));
#15103=DIRECTION('',(0.,0.,1.));
#15104=DIRECTION('',(0.,0.,1.));
#15105=DIRECTION('',(-1.,0.,0.));
#15106=DIRECTION('center_axis',(-1.,0.,0.));
#15107=DIRECTION('ref_axis',(0.,1.,0.));
#15108=DIRECTION('center_axis',(1.,0.,0.));
#15109=DIRECTION('ref_axis',(0.,1.,0.));
#15110=DIRECTION('center_axis',(1.,0.,0.));
#15111=DIRECTION('ref_axis',(0.,1.,0.));
#15112=DIRECTION('center_axis',(-1.,0.,0.));
#15113=DIRECTION('ref_axis',(0.,-1.,0.));
#15114=DIRECTION('center_axis',(1.,0.,0.));
#15115=DIRECTION('ref_axis',(0.,-1.,0.));
#15116=DIRECTION('',(-1.,0.,0.));
#15117=DIRECTION('center_axis',(1.,0.,0.));
#15118=DIRECTION('ref_axis',(0.,-1.,0.));
#15119=DIRECTION('center_axis',(-1.,0.,0.));
#15120=DIRECTION('ref_axis',(0.,-1.,0.));
#15121=DIRECTION('center_axis',(1.,0.,0.));
#15122=DIRECTION('ref_axis',(0.,-1.,0.));
#15123=DIRECTION('',(-1.,0.,0.));
#15124=DIRECTION('center_axis',(1.,0.,0.));
#15125=DIRECTION('ref_axis',(0.,-1.,0.));
#15126=DIRECTION('center_axis',(0.,1.49175803335835E-16,-1.));
#15127=DIRECTION('ref_axis',(0.,-1.,-1.49175803335835E-16));
#15128=DIRECTION('',(0.,1.,1.49175803335835E-16));
#15129=DIRECTION('',(-1.,0.,0.));
#15130=DIRECTION('',(0.,-1.,-1.49175803335835E-16));
#15131=DIRECTION('',(-1.,0.,0.));
#15132=DIRECTION('center_axis',(-1.,0.,0.));
#15133=DIRECTION('ref_axis',(0.,1.,-1.18423789293348E-14));
#15134=DIRECTION('center_axis',(-1.,0.,0.));
#15135=DIRECTION('ref_axis',(0.,1.,-1.18423789293348E-14));
#15136=DIRECTION('center_axis',(-1.,0.,0.));
#15137=DIRECTION('ref_axis',(0.,1.,-1.18423789293348E-14));
#15138=DIRECTION('',(-1.,0.,0.));
#15139=DIRECTION('center_axis',(0.,1.,0.));
#15140=DIRECTION('ref_axis',(0.,0.,-1.));
#15141=DIRECTION('',(0.,0.,1.));
#15142=DIRECTION('',(0.,0.,-1.));
#15143=DIRECTION('',(-1.,0.,0.));
#15144=DIRECTION('center_axis',(-1.,0.,0.));
#15145=DIRECTION('ref_axis',(0.,1.18423789293349E-14,1.));
#15146=DIRECTION('center_axis',(-1.,0.,0.));
#15147=DIRECTION('ref_axis',(0.,1.18423789293349E-14,1.));
#15148=DIRECTION('center_axis',(-1.,0.,0.));
#15149=DIRECTION('ref_axis',(0.,1.18423789293349E-14,1.));
#15150=DIRECTION('',(-1.,0.,0.));
#15151=DIRECTION('center_axis',(0.,0.,1.));
#15152=DIRECTION('ref_axis',(0.,1.,0.));
#15153=DIRECTION('',(0.,-1.,0.));
#15154=DIRECTION('',(0.,1.,0.));
#15155=DIRECTION('',(-1.,0.,0.));
#15156=DIRECTION('center_axis',(-1.,0.,0.));
#15157=DIRECTION('ref_axis',(0.,-1.,1.18423789293348E-14));
#15158=DIRECTION('center_axis',(-1.,0.,0.));
#15159=DIRECTION('ref_axis',(0.,-1.,1.18423789293348E-14));
#15160=DIRECTION('center_axis',(-1.,0.,0.));
#15161=DIRECTION('ref_axis',(0.,-1.,1.18423789293348E-14));
#15162=DIRECTION('',(-1.,0.,0.));
#15163=DIRECTION('center_axis',(0.,-1.,0.));
#15164=DIRECTION('ref_axis',(0.,0.,1.));
#15165=DIRECTION('',(0.,0.,-1.));
#15166=DIRECTION('',(0.,0.,1.));
#15167=DIRECTION('',(-1.,0.,0.));
#15168=DIRECTION('center_axis',(-1.,0.,0.));
#15169=DIRECTION('ref_axis',(0.,-1.18423789293348E-14,-1.));
#15170=DIRECTION('center_axis',(-1.,0.,0.));
#15171=DIRECTION('ref_axis',(0.,-1.18423789293348E-14,-1.));
#15172=DIRECTION('center_axis',(-1.,0.,0.));
#15173=DIRECTION('ref_axis',(0.,-1.18423789293348E-14,-1.));
#15174=DIRECTION('center_axis',(-1.,0.,0.));
#15175=DIRECTION('ref_axis',(0.,-1.,0.));
#15176=DIRECTION('center_axis',(-1.,0.,0.));
#15177=DIRECTION('ref_axis',(0.,-1.,0.));
#35926=CARTESIAN_POINT('',(0.,0.,0.));
#35927=CARTESIAN_POINT('Origin',(-22.5,232.431902763327,-19.1700672509895));
#35928=CARTESIAN_POINT('',(-22.5,234.931902763327,-19.1700672509895));
#35929=CARTESIAN_POINT('Origin',(-22.5,232.431902763327,-19.1700672509895));
#35930=CARTESIAN_POINT('',(-24.5,234.931902763327,-19.1700672509894));
#35931=CARTESIAN_POINT('',(-22.5,234.931902763327,-19.1700672509895));
#35932=CARTESIAN_POINT('Origin',(-24.5,232.431902763327,-19.1700672509895));
#35933=CARTESIAN_POINT('Origin',(-22.5,182.525945920127,23.982775519786));
#35934=CARTESIAN_POINT('',(-22.5,182.525945920127,23.982775519786));
#35935=CARTESIAN_POINT('',(-22.5,182.525945920127,17.2567109421317));
#35936=CARTESIAN_POINT('',(-22.5,182.525945920127,17.2567109421317));
#35937=CARTESIAN_POINT('',(-24.5,182.525945920127,17.2567109421317));
#35938=CARTESIAN_POINT('',(-22.5,182.525945920127,17.2567109421317));
#35939=CARTESIAN_POINT('',(-24.5,182.525945920127,23.982775519786));
#35940=CARTESIAN_POINT('',(-24.5,182.525945920127,17.2567109421317));
#35941=CARTESIAN_POINT('',(-22.5,182.525945920127,23.982775519786));
#35942=CARTESIAN_POINT('Origin',(-22.5,183.91845147722,23.982775519786));
#35943=CARTESIAN_POINT('',(-22.5,185.310957034312,23.982775519786));
#35944=CARTESIAN_POINT('Origin',(-22.5,183.91845147722,23.982775519786));
#35945=CARTESIAN_POINT('',(-24.5,185.310957034312,23.982775519786));
#35946=CARTESIAN_POINT('Origin',(-24.5,183.91845147722,23.982775519786));
#35947=CARTESIAN_POINT('',(-22.5,185.310957034312,23.982775519786));
#35948=CARTESIAN_POINT('Origin',(-22.5,185.310957034312,17.2567109421317));
#35949=CARTESIAN_POINT('',(-22.5,185.310957034312,17.2567109421317));
#35950=CARTESIAN_POINT('',(-22.5,185.310957034312,23.982775519786));
#35951=CARTESIAN_POINT('',(-24.5,185.310957034312,17.2567109421317));
#35952=CARTESIAN_POINT('',(-24.5,185.310957034312,23.982775519786));
#35953=CARTESIAN_POINT('',(-22.5,185.310957034312,17.2567109421317));
#35954=CARTESIAN_POINT('Origin',(-22.5,183.91845147722,17.2567109421317));
#35955=CARTESIAN_POINT('Origin',(-22.5,183.91845147722,17.2567109421317));
#35956=CARTESIAN_POINT('Origin',(-24.5,183.91845147722,17.2567109421317));
#35957=CARTESIAN_POINT('Origin',(-22.5,211.657861025925,0.886420913981472));
#35958=CARTESIAN_POINT('',(-22.5,214.124612099013,0.886420913981471));
#35959=CARTESIAN_POINT('Origin',(-22.5,211.657861025925,0.886420913981472));
#35960=CARTESIAN_POINT('',(-24.5,214.124612099013,0.886420913981472));
#35961=CARTESIAN_POINT('',(-22.5,214.124612099013,0.886420913981472));
#35962=CARTESIAN_POINT('Origin',(-24.5,211.657861025925,0.886420913981472));
#35963=CARTESIAN_POINT('Origin',(-22.5,221.602473620571,-19.1135790860185));
#35964=CARTESIAN_POINT('',(-22.5,224.069224693659,-19.1135790860185));
#35965=CARTESIAN_POINT('Origin',(-22.5,221.602473620571,-19.1135790860185));
#35966=CARTESIAN_POINT('',(-24.5,224.069224693659,-19.1135790860185));
#35967=CARTESIAN_POINT('',(-22.5,224.069224693659,-19.1135790860185));
#35968=CARTESIAN_POINT('Origin',(-24.5,221.602473620571,-19.1135790860185));
#35969=CARTESIAN_POINT('Origin',(-22.5,211.657861025925,-19.1135790860185));
#35970=CARTESIAN_POINT('',(-22.5,214.124612099013,-19.1135790860185));
#35971=CARTESIAN_POINT('Origin',(-22.5,211.657861025925,-19.1135790860185));
#35972=CARTESIAN_POINT('',(-24.5,214.124612099013,-19.1135790860185));
#35973=CARTESIAN_POINT('',(-22.5,214.124612099013,-19.1135790860185));
#35974=CARTESIAN_POINT('Origin',(-24.5,211.657861025925,-19.1135790860185));
#35975=CARTESIAN_POINT('Origin',(-22.5,211.657861025925,20.8864209139815));
#35976=CARTESIAN_POINT('',(-22.5,214.124612099013,20.8864209139815));
#35977=CARTESIAN_POINT('Origin',(-22.5,211.657861025925,20.8864209139815));
#35978=CARTESIAN_POINT('',(-24.5,214.124612099013,20.8864209139815));
#35979=CARTESIAN_POINT('',(-22.5,214.124612099013,20.8864209139815));
#35980=CARTESIAN_POINT('Origin',(-24.5,211.657861025925,20.8864209139815));
#35981=CARTESIAN_POINT('Origin',(-22.5,201.657861025925,20.8864209139815));
#35982=CARTESIAN_POINT('',(-22.5,204.124612099013,20.8864209139815));
#35983=CARTESIAN_POINT('Origin',(-22.5,201.657861025925,20.8864209139815));
#35984=CARTESIAN_POINT('',(-24.5,204.124612099013,20.8864209139815));
#35985=CARTESIAN_POINT('',(-22.5,204.124612099013,20.8864209139815));
#35986=CARTESIAN_POINT('Origin',(-24.5,201.657861025925,20.8864209139815));
#35987=CARTESIAN_POINT('Origin',(-22.5,189.00788651778,10.7107295366928));
#35988=CARTESIAN_POINT('',(-22.5,189.00788651778,10.7107295366928));
#35989=CARTESIAN_POINT('',(-22.5,189.00788651778,-9.36247421041762));
#35990=CARTESIAN_POINT('',(-22.5,189.00788651778,-9.36247421041762));
#35991=CARTESIAN_POINT('',(-24.5,189.00788651778,-9.36247421041762));
#35992=CARTESIAN_POINT('',(-22.5,189.00788651778,-9.36247421041762));
#35993=CARTESIAN_POINT('',(-24.5,189.00788651778,10.7107295366928));
#35994=CARTESIAN_POINT('',(-24.5,189.00788651778,-9.36247421041762));
#35995=CARTESIAN_POINT('',(-22.5,189.00788651778,10.7107295366928));
#35996=CARTESIAN_POINT('Origin',(-22.5,191.707791115344,10.7107295366928));
#35997=CARTESIAN_POINT('',(-22.5,194.407695712909,10.7107295366928));
#35998=CARTESIAN_POINT('Origin',(-22.5,191.707791115344,10.7107295366928));
#35999=CARTESIAN_POINT('',(-24.5,194.407695712909,10.7107295366928));
#36000=CARTESIAN_POINT('Origin',(-24.5,191.707791115344,10.7107295366928));
#36001=CARTESIAN_POINT('',(-22.5,194.407695712909,10.7107295366928));
#36002=CARTESIAN_POINT('Origin',(-22.5,194.407695712909,-9.36247421041762));
#36003=CARTESIAN_POINT('',(-22.5,194.407695712909,-9.36247421041762));
#36004=CARTESIAN_POINT('',(-22.5,194.407695712909,10.7107295366928));
#36005=CARTESIAN_POINT('',(-24.5,194.407695712909,-9.36247421041762));
#36006=CARTESIAN_POINT('',(-24.5,194.407695712909,10.7107295366928));
#36007=CARTESIAN_POINT('',(-22.5,194.407695712909,-9.36247421041762));
#36008=CARTESIAN_POINT('Origin',(-22.5,191.707791115344,-9.36247421041762));
#36009=CARTESIAN_POINT('Origin',(-22.5,191.707791115344,-9.36247421041762));
#36010=CARTESIAN_POINT('Origin',(-24.5,191.707791115344,-9.36247421041762));
#36011=CARTESIAN_POINT('Origin',(-22.5,237.949377612184,-16.017224480214));
#36012=CARTESIAN_POINT('',(-22.5,237.949377612184,-16.017224480214));
#36013=CARTESIAN_POINT('',(-22.5,237.949377612184,-22.7432890578683));
#36014=CARTESIAN_POINT('',(-22.5,237.949377612184,-16.017224480214));
#36015=CARTESIAN_POINT('',(-24.5,237.949377612184,-22.7432890578683));
#36016=CARTESIAN_POINT('',(-22.5,237.949377612184,-22.7432890578683));
#36017=CARTESIAN_POINT('',(-24.5,237.949377612184,-16.017224480214));
#36018=CARTESIAN_POINT('',(-24.5,237.949377612184,-16.017224480214));
#36019=CARTESIAN_POINT('',(-22.5,237.949377612184,-16.017224480214));
#36020=CARTESIAN_POINT('Origin',(-22.5,239.341883169277,-16.017224480214));
#36021=CARTESIAN_POINT('',(-22.5,240.734388726369,-16.017224480214));
#36022=CARTESIAN_POINT('Origin',(-22.5,239.341883169277,-16.017224480214));
#36023=CARTESIAN_POINT('',(-24.5,240.734388726369,-16.017224480214));
#36024=CARTESIAN_POINT('Origin',(-24.5,239.341883169277,-16.017224480214));
#36025=CARTESIAN_POINT('',(-22.5,240.734388726369,-16.017224480214));
#36026=CARTESIAN_POINT('Origin',(-22.5,240.734388726369,-22.7432890578683));
#36027=CARTESIAN_POINT('',(-22.5,240.734388726369,-22.7432890578683));
#36028=CARTESIAN_POINT('',(-22.5,240.734388726369,-22.7432890578683));
#36029=CARTESIAN_POINT('',(-24.5,240.734388726369,-22.7432890578683));
#36030=CARTESIAN_POINT('',(-24.5,240.734388726369,-22.7432890578683));
#36031=CARTESIAN_POINT('',(-22.5,240.734388726369,-22.7432890578683));
#36032=CARTESIAN_POINT('Origin',(-22.5,239.341883169277,-22.7432890578683));
#36033=CARTESIAN_POINT('Origin',(-22.5,239.341883169277,-22.7432890578683));
#36034=CARTESIAN_POINT('Origin',(-24.5,239.341883169277,-22.7432890578683));
#36035=CARTESIAN_POINT('Origin',(-22.5,190.828431883169,-19.1700672509895));
#36036=CARTESIAN_POINT('',(-22.5,193.328431883169,-19.1700672509895));
#36037=CARTESIAN_POINT('Origin',(-22.5,190.828431883169,-19.1700672509895));
#36038=CARTESIAN_POINT('',(-24.5,193.328431883169,-19.1700672509894));
#36039=CARTESIAN_POINT('',(-22.5,193.328431883169,-19.1700672509895));
#36040=CARTESIAN_POINT('Origin',(-24.5,190.828431883169,-19.1700672509895));
#36041=CARTESIAN_POINT('Origin',(-22.5,221.602473620571,0.886420913981474));
#36042=CARTESIAN_POINT('',(-22.5,224.069224693659,0.886420913981474));
#36043=CARTESIAN_POINT('Origin',(-22.5,221.602473620571,0.886420913981474));
#36044=CARTESIAN_POINT('',(-24.5,224.069224693659,0.886420913981474));
#36045=CARTESIAN_POINT('',(-22.5,224.069224693659,0.886420913981474));
#36046=CARTESIAN_POINT('Origin',(-24.5,221.602473620571,0.886420913981474));
#36047=CARTESIAN_POINT('Origin',(-22.5,190.828431883169,20.8299327490105));
#36048=CARTESIAN_POINT('',(-22.5,193.328431883169,20.8299327490105));
#36049=CARTESIAN_POINT('Origin',(-22.5,190.828431883169,20.8299327490105));
#36050=CARTESIAN_POINT('',(-24.5,193.328431883169,20.8299327490105));
#36051=CARTESIAN_POINT('',(-22.5,193.328431883169,20.8299327490105));
#36052=CARTESIAN_POINT('Origin',(-24.5,190.828431883169,20.8299327490105));
#36053=CARTESIAN_POINT('Origin',(-22.5,201.657861025925,0.886420913981472));
#36054=CARTESIAN_POINT('',(-22.5,204.124612099013,0.886420913981471));
#36055=CARTESIAN_POINT('Origin',(-22.5,201.657861025925,0.886420913981472));
#36056=CARTESIAN_POINT('',(-24.5,204.124612099013,0.886420913981472));
#36057=CARTESIAN_POINT('',(-22.5,204.124612099013,0.886420913981472));
#36058=CARTESIAN_POINT('Origin',(-24.5,201.657861025925,0.886420913981472));
#36059=CARTESIAN_POINT('Origin',(-22.5,201.657861025925,-19.1135790860185));
#36060=CARTESIAN_POINT('',(-22.5,204.124612099013,-19.1135790860185));
#36061=CARTESIAN_POINT('Origin',(-22.5,201.657861025925,-19.1135790860185));
#36062=CARTESIAN_POINT('',(-24.5,204.124612099013,-19.1135790860185));
#36063=CARTESIAN_POINT('',(-22.5,204.124612099013,-19.1135790860185));
#36064=CARTESIAN_POINT('Origin',(-24.5,201.657861025925,-19.1135790860185));
#36065=CARTESIAN_POINT('Origin',(-22.5,185.310957034312,-2.74328905786827));
#36066=CARTESIAN_POINT('',(-22.5,185.310957034312,-2.74328905786827));
#36067=CARTESIAN_POINT('',(-22.5,185.310957034312,3.98277551978598));
#36068=CARTESIAN_POINT('',(-22.5,185.310957034312,3.98277551978598));
#36069=CARTESIAN_POINT('',(-24.5,185.310957034312,3.98277551978598));
#36070=CARTESIAN_POINT('',(-22.5,185.310957034312,3.98277551978598));
#36071=CARTESIAN_POINT('',(-24.5,185.310957034312,-2.74328905786827));
#36072=CARTESIAN_POINT('',(-24.5,185.310957034312,3.98277551978598));
#36073=CARTESIAN_POINT('',(-22.5,185.310957034312,-2.74328905786827));
#36074=CARTESIAN_POINT('Origin',(-22.5,183.91845147722,-2.74328905786827));
#36075=CARTESIAN_POINT('',(-22.5,182.525945920127,-2.74328905786827));
#36076=CARTESIAN_POINT('Origin',(-22.5,183.91845147722,-2.74328905786827));
#36077=CARTESIAN_POINT('',(-24.5,182.525945920127,-2.74328905786827));
#36078=CARTESIAN_POINT('Origin',(-24.5,183.91845147722,-2.74328905786827));
#36079=CARTESIAN_POINT('',(-22.5,182.525945920127,-2.74328905786827));
#36080=CARTESIAN_POINT('Origin',(-22.5,182.525945920127,3.98277551978598));
#36081=CARTESIAN_POINT('',(-22.5,182.525945920127,3.98277551978598));
#36082=CARTESIAN_POINT('',(-22.5,182.525945920127,-2.74328905786827));
#36083=CARTESIAN_POINT('',(-24.5,182.525945920127,3.98277551978598));
#36084=CARTESIAN_POINT('',(-24.5,182.525945920127,-2.74328905786827));
#36085=CARTESIAN_POINT('',(-22.5,182.525945920127,3.98277551978598));
#36086=CARTESIAN_POINT('Origin',(-22.5,183.91845147722,3.98277551978598));
#36087=CARTESIAN_POINT('Origin',(-22.5,183.91845147722,3.98277551978598));
#36088=CARTESIAN_POINT('Origin',(-24.5,183.91845147722,3.98277551978598));
#36089=CARTESIAN_POINT('Origin',(-22.5,232.431902763327,20.8299327490105));
#36090=CARTESIAN_POINT('',(-22.5,234.931902763327,20.8299327490105));
#36091=CARTESIAN_POINT('Origin',(-22.5,232.431902763327,20.8299327490105));
#36092=CARTESIAN_POINT('',(-24.5,234.931902763327,20.8299327490105));
#36093=CARTESIAN_POINT('',(-22.5,234.931902763327,20.8299327490105));
#36094=CARTESIAN_POINT('Origin',(-24.5,232.431902763327,20.8299327490105));
#36095=CARTESIAN_POINT('Origin',(-22.5,221.602473620571,20.8864209139815));
#36096=CARTESIAN_POINT('',(-22.5,224.069224693659,20.8864209139815));
#36097=CARTESIAN_POINT('Origin',(-22.5,221.602473620571,20.8864209139815));
#36098=CARTESIAN_POINT('',(-24.5,224.069224693659,20.8864209139815));
#36099=CARTESIAN_POINT('',(-22.5,224.069224693659,20.8864209139815));
#36100=CARTESIAN_POINT('Origin',(-24.5,221.602473620571,20.8864209139815));
#36101=CARTESIAN_POINT('Origin',(-22.5,237.949377612184,3.98277551978598));
#36102=CARTESIAN_POINT('',(-22.5,237.949377612184,3.98277551978598));
#36103=CARTESIAN_POINT('',(-22.5,237.949377612184,-2.74328905786827));
#36104=CARTESIAN_POINT('',(-22.5,237.949377612184,3.98277551978598));
#36105=CARTESIAN_POINT('',(-24.5,237.949377612184,-2.74328905786827));
#36106=CARTESIAN_POINT('',(-22.5,237.949377612184,-2.74328905786827));
#36107=CARTESIAN_POINT('',(-24.5,237.949377612184,3.98277551978598));
#36108=CARTESIAN_POINT('',(-24.5,237.949377612184,3.98277551978598));
#36109=CARTESIAN_POINT('',(-22.5,237.949377612184,3.98277551978598));
#36110=CARTESIAN_POINT('Origin',(-22.5,239.341883169277,3.98277551978598));
#36111=CARTESIAN_POINT('',(-22.5,240.734388726369,3.98277551978598));
#36112=CARTESIAN_POINT('Origin',(-22.5,239.341883169277,3.98277551978598));
#36113=CARTESIAN_POINT('',(-24.5,240.734388726369,3.98277551978598));
#36114=CARTESIAN_POINT('Origin',(-24.5,239.341883169277,3.98277551978598));
#36115=CARTESIAN_POINT('',(-22.5,240.734388726369,3.98277551978598));
#36116=CARTESIAN_POINT('Origin',(-22.5,240.734388726369,-2.74328905786827));
#36117=CARTESIAN_POINT('',(-22.5,240.734388726369,-2.74328905786827));
#36118=CARTESIAN_POINT('',(-22.5,240.734388726369,-2.74328905786827));
#36119=CARTESIAN_POINT('',(-24.5,240.734388726369,-2.74328905786827));
#36120=CARTESIAN_POINT('',(-24.5,240.734388726369,-2.74328905786827));
#36121=CARTESIAN_POINT('',(-22.5,240.734388726369,-2.74328905786827));
#36122=CARTESIAN_POINT('Origin',(-22.5,239.341883169277,-2.74328905786827));
#36123=CARTESIAN_POINT('Origin',(-22.5,239.341883169277,-2.74328905786827));
#36124=CARTESIAN_POINT('Origin',(-24.5,239.341883169277,-2.74328905786827));
#36125=CARTESIAN_POINT('Origin',(-22.5,185.310957034312,-22.7432890578683));
#36126=CARTESIAN_POINT('',(-22.5,185.310957034312,-22.7432890578683));
#36127=CARTESIAN_POINT('',(-22.5,185.310957034312,-16.017224480214));
#36128=CARTESIAN_POINT('',(-22.5,185.310957034312,-16.017224480214));
#36129=CARTESIAN_POINT('',(-24.5,185.310957034312,-16.017224480214));
#36130=CARTESIAN_POINT('',(-22.5,185.310957034312,-16.017224480214));
#36131=CARTESIAN_POINT('',(-24.5,185.310957034312,-22.7432890578683));
#36132=CARTESIAN_POINT('',(-24.5,185.310957034312,-16.017224480214));
#36133=CARTESIAN_POINT('',(-22.5,185.310957034312,-22.7432890578683));
#36134=CARTESIAN_POINT('Origin',(-22.5,183.91845147722,-22.7432890578683));
#36135=CARTESIAN_POINT('',(-22.5,182.525945920127,-22.7432890578683));
#36136=CARTESIAN_POINT('Origin',(-22.5,183.91845147722,-22.7432890578683));
#36137=CARTESIAN_POINT('',(-24.5,182.525945920127,-22.7432890578683));
#36138=CARTESIAN_POINT('Origin',(-24.5,183.91845147722,-22.7432890578683));
#36139=CARTESIAN_POINT('',(-22.5,182.525945920127,-22.7432890578683));
#36140=CARTESIAN_POINT('Origin',(-22.5,182.525945920127,-16.017224480214));
#36141=CARTESIAN_POINT('',(-22.5,182.525945920127,-16.017224480214));
#36142=CARTESIAN_POINT('',(-22.5,182.525945920127,-22.7432890578683));
#36143=CARTESIAN_POINT('',(-24.5,182.525945920127,-16.017224480214));
#36144=CARTESIAN_POINT('',(-24.5,182.525945920127,-22.7432890578683));
#36145=CARTESIAN_POINT('',(-22.5,182.525945920127,-16.017224480214));
#36146=CARTESIAN_POINT('Origin',(-22.5,183.91845147722,-16.017224480214));
#36147=CARTESIAN_POINT('Origin',(-22.5,183.91845147722,-16.017224480214));
#36148=CARTESIAN_POINT('Origin',(-24.5,183.91845147722,-16.017224480214));
#36149=CARTESIAN_POINT('Origin',(-22.5,237.949377612184,23.982775519786));
#36150=CARTESIAN_POINT('',(-22.5,237.949377612184,23.982775519786));
#36151=CARTESIAN_POINT('',(-22.5,237.949377612184,17.2567109421317));
#36152=CARTESIAN_POINT('',(-22.5,237.949377612184,23.982775519786));
#36153=CARTESIAN_POINT('',(-24.5,237.949377612184,17.2567109421317));
#36154=CARTESIAN_POINT('',(-22.5,237.949377612184,17.2567109421317));
#36155=CARTESIAN_POINT('',(-24.5,237.949377612184,23.982775519786));
#36156=CARTESIAN_POINT('',(-24.5,237.949377612184,23.982775519786));
#36157=CARTESIAN_POINT('',(-22.5,237.949377612184,23.982775519786));
#36158=CARTESIAN_POINT('Origin',(-22.5,239.341883169277,23.982775519786));
#36159=CARTESIAN_POINT('',(-22.5,240.734388726369,23.982775519786));
#36160=CARTESIAN_POINT('Origin',(-22.5,239.341883169277,23.982775519786));
#36161=CARTESIAN_POINT('',(-24.5,240.734388726369,23.982775519786));
#36162=CARTESIAN_POINT('Origin',(-24.5,239.341883169277,23.982775519786));
#36163=CARTESIAN_POINT('',(-22.5,240.734388726369,23.982775519786));
#36164=CARTESIAN_POINT('Origin',(-22.5,240.734388726369,17.2567109421317));
#36165=CARTESIAN_POINT('',(-22.5,240.734388726369,17.2567109421317));
#36166=CARTESIAN_POINT('',(-22.5,240.734388726369,17.2567109421317));
#36167=CARTESIAN_POINT('',(-24.5,240.734388726369,17.2567109421317));
#36168=CARTESIAN_POINT('',(-24.5,240.734388726369,17.2567109421317));
#36169=CARTESIAN_POINT('',(-22.5,240.734388726369,17.2567109421317));
#36170=CARTESIAN_POINT('Origin',(-22.5,239.341883169277,17.2567109421317));
#36171=CARTESIAN_POINT('Origin',(-22.5,239.341883169277,17.2567109421317));
#36172=CARTESIAN_POINT('Origin',(-24.5,239.341883169277,17.2567109421317));
#36173=CARTESIAN_POINT('Origin',(-22.5,228.852638933588,10.7107295366928));
#36174=CARTESIAN_POINT('',(-22.5,228.852638933588,10.7107295366928));
#36175=CARTESIAN_POINT('',(-22.5,228.852638933588,-9.36247421041762));
#36176=CARTESIAN_POINT('',(-22.5,228.852638933588,10.7107295366928));
#36177=CARTESIAN_POINT('',(-24.5,228.852638933588,-9.36247421041762));
#36178=CARTESIAN_POINT('',(-22.5,228.852638933588,-9.36247421041762));
#36179=CARTESIAN_POINT('',(-24.5,228.852638933588,10.7107295366928));
#36180=CARTESIAN_POINT('',(-24.5,228.852638933588,10.7107295366928));
#36181=CARTESIAN_POINT('',(-22.5,228.852638933588,10.7107295366928));
#36182=CARTESIAN_POINT('Origin',(-22.5,231.552543531152,10.7107295366928));
#36183=CARTESIAN_POINT('',(-22.5,234.252448128717,10.7107295366928));
#36184=CARTESIAN_POINT('Origin',(-22.5,231.552543531152,10.7107295366928));
#36185=CARTESIAN_POINT('',(-24.5,234.252448128717,10.7107295366928));
#36186=CARTESIAN_POINT('Origin',(-24.5,231.552543531152,10.7107295366928));
#36187=CARTESIAN_POINT('',(-22.5,234.252448128717,10.7107295366928));
#36188=CARTESIAN_POINT('Origin',(-22.5,234.252448128717,-9.36247421041762));
#36189=CARTESIAN_POINT('',(-22.5,234.252448128717,-9.36247421041762));
#36190=CARTESIAN_POINT('',(-22.5,234.252448128717,-9.36247421041762));
#36191=CARTESIAN_POINT('',(-24.5,234.252448128717,-9.36247421041762));
#36192=CARTESIAN_POINT('',(-24.5,234.252448128717,-9.36247421041762));
#36193=CARTESIAN_POINT('',(-22.5,234.252448128717,-9.36247421041762));
#36194=CARTESIAN_POINT('Origin',(-22.5,231.552543531152,-9.36247421041762));
#36195=CARTESIAN_POINT('Origin',(-22.5,231.552543531152,-9.36247421041762));
#36196=CARTESIAN_POINT('Origin',(-24.5,231.552543531152,-9.36247421041762));
#36197=CARTESIAN_POINT('Origin',(-22.5,211.657861025925,-9.11357908601853));
#36198=CARTESIAN_POINT('',(-22.5,214.124612099013,-9.11357908601853));
#36199=CARTESIAN_POINT('Origin',(-22.5,211.657861025925,-9.11357908601853));
#36200=CARTESIAN_POINT('',(-24.5,214.124612099013,-9.11357908601853));
#36201=CARTESIAN_POINT('',(-22.5,214.124612099013,-9.11357908601853));
#36202=CARTESIAN_POINT('Origin',(-24.5,211.657861025925,-9.11357908601853));
#36203=CARTESIAN_POINT('Origin',(-22.5,211.657861025925,10.8864209139815));
#36204=CARTESIAN_POINT('',(-22.5,214.124612099013,10.8864209139815));
#36205=CARTESIAN_POINT('Origin',(-22.5,211.657861025925,10.8864209139815));
#36206=CARTESIAN_POINT('',(-24.5,214.124612099013,10.8864209139815));
#36207=CARTESIAN_POINT('',(-22.5,214.124612099013,10.8864209139815));
#36208=CARTESIAN_POINT('Origin',(-24.5,211.657861025925,10.8864209139815));
#36209=CARTESIAN_POINT('Origin',(-22.5,241.399687575155,-32.0121872517985));
#36210=CARTESIAN_POINT('',(-22.5,181.860647071341,-32.0121872517985));
#36211=CARTESIAN_POINT('',(-22.5,241.399687575155,-32.0121872517985));
#36212=CARTESIAN_POINT('',(-22.5,181.860647071341,-32.0121872517985));
#36213=CARTESIAN_POINT('',(-24.5,181.860647071341,-32.0121872517985));
#36214=CARTESIAN_POINT('',(-22.5,181.860647071341,-32.0121872517985));
#36215=CARTESIAN_POINT('',(-24.5,241.399687575155,-32.0121872517985));
#36216=CARTESIAN_POINT('',(-24.5,181.860647071341,-32.0121872517985));
#36217=CARTESIAN_POINT('',(-22.5,241.399687575155,-32.0121872517985));
#36218=CARTESIAN_POINT('Origin',(-22.5,241.399687575155,-29.0121872517985));
#36219=CARTESIAN_POINT('',(-22.5,244.399687575155,-29.0121872517985));
#36220=CARTESIAN_POINT('Origin',(-22.5,241.399687575155,-29.0121872517985));
#36221=CARTESIAN_POINT('',(-24.5,244.399687575155,-29.0121872517985));
#36222=CARTESIAN_POINT('Origin',(-24.5,241.399687575155,-29.0121872517985));
#36223=CARTESIAN_POINT('',(-22.5,244.399687575155,-29.0121872517985));
#36224=CARTESIAN_POINT('Origin',(-22.5,244.399687575155,30.5413729944905));
#36225=CARTESIAN_POINT('',(-22.5,244.399687575155,30.5413729944905));
#36226=CARTESIAN_POINT('',(-22.5,244.399687575155,-29.0121872517985));
#36227=CARTESIAN_POINT('',(-24.5,244.399687575155,30.5413729944905));
#36228=CARTESIAN_POINT('',(-24.5,244.399687575155,-29.0121872517985));
#36229=CARTESIAN_POINT('',(-22.5,244.399687575155,30.5413729944905));
#36230=CARTESIAN_POINT('Origin',(-22.5,241.399687575155,30.5413729944905));
#36231=CARTESIAN_POINT('',(-22.5,241.399687575155,33.5413729944905));
#36232=CARTESIAN_POINT('Origin',(-22.5,241.399687575155,30.5413729944905));
#36233=CARTESIAN_POINT('',(-24.5,241.399687575155,33.5413729944905));
#36234=CARTESIAN_POINT('Origin',(-24.5,241.399687575155,30.5413729944905));
#36235=CARTESIAN_POINT('',(-22.5,241.399687575155,33.5413729944905));
#36236=CARTESIAN_POINT('Origin',(-22.5,181.860647071341,33.5413729944905));
#36237=CARTESIAN_POINT('',(-22.5,181.860647071341,33.5413729944905));
#36238=CARTESIAN_POINT('',(-22.5,241.399687575155,33.5413729944905));
#36239=CARTESIAN_POINT('',(-24.5,181.860647071341,33.5413729944905));
#36240=CARTESIAN_POINT('',(-24.5,241.399687575155,33.5413729944905));
#36241=CARTESIAN_POINT('',(-22.5,181.860647071341,33.5413729944905));
#36242=CARTESIAN_POINT('Origin',(-22.5,181.860647071341,30.5413729944905));
#36243=CARTESIAN_POINT('',(-22.5,178.860647071341,30.5413729944905));
#36244=CARTESIAN_POINT('Origin',(-22.5,181.860647071341,30.5413729944905));
#36245=CARTESIAN_POINT('',(-24.5,178.860647071341,30.5413729944905));
#36246=CARTESIAN_POINT('Origin',(-24.5,181.860647071341,30.5413729944905));
#36247=CARTESIAN_POINT('',(-22.5,178.860647071341,30.5413729944905));
#36248=CARTESIAN_POINT('Origin',(-22.5,178.860647071341,-29.0121872517985));
#36249=CARTESIAN_POINT('',(-22.5,178.860647071341,-29.0121872517985));
#36250=CARTESIAN_POINT('',(-22.5,178.860647071341,30.5413729944905));
#36251=CARTESIAN_POINT('',(-24.5,178.860647071341,-29.0121872517985));
#36252=CARTESIAN_POINT('',(-24.5,178.860647071341,30.5413729944905));
#36253=CARTESIAN_POINT('',(-22.5,178.860647071341,-29.0121872517985));
#36254=CARTESIAN_POINT('Origin',(-22.5,181.860647071341,-29.0121872517985));
#36255=CARTESIAN_POINT('Origin',(-22.5,181.860647071341,-29.0121872517985));
#36256=CARTESIAN_POINT('Origin',(-24.5,181.860647071341,-29.0121872517985));
#36257=CARTESIAN_POINT('Origin',(-24.5,211.630167323248,0.764592871346017));
#36258=CARTESIAN_POINT('Origin',(-22.5,211.630167323248,0.764592871346017));
#36441=UNCERTAINTY_MEASURE_WITH_UNIT(LENGTH_MEASURE(0.01),#36461,
'DISTANCE_ACCURACY_VALUE',
'Maximum model space distance between geometric entities at asserted c
onnectivities');
#36444=UNCERTAINTY_MEASURE_WITH_UNIT(LENGTH_MEASURE(0.01),#36461,
'DISTANCE_ACCURACY_VALUE',
'Maximum model space distance between geometric entities at asserted c
onnectivities');
#36457=(
GEOMETRIC_REPRESENTATION_CONTEXT(3)
GLOBAL_UNCERTAINTY_ASSIGNED_CONTEXT((#36441))
GLOBAL_UNIT_ASSIGNED_CONTEXT((#36461,#36463,#36464))
REPRESENTATION_CONTEXT('','3D')
);
#36460=(
GEOMETRIC_REPRESENTATION_CONTEXT(3)
GLOBAL_UNCERTAINTY_ASSIGNED_CONTEXT((#36444))
GLOBAL_UNIT_ASSIGNED_CONTEXT((#36461,#36463,#36464))
REPRESENTATION_CONTEXT('','3D')
);
#36461=(
LENGTH_UNIT()
NAMED_UNIT(*)
SI_UNIT(.MILLI.,.METRE.)
);
#36463=(
NAMED_UNIT(*)
PLANE_ANGLE_UNIT()
SI_UNIT($,.RADIAN.)
);
#36464=(
NAMED_UNIT(*)
SI_UNIT($,.STERADIAN.)
SOLID_ANGLE_UNIT()
);
#36477=SHAPE_DEFINITION_REPRESENTATION(#36497,#36528);
#36497=PRODUCT_DEFINITION_SHAPE('',$,#36544);
#36528=SHAPE_REPRESENTATION('',(#12231),#36457);
#36531=PRODUCT_DEFINITION_CONTEXT('part definition',#36578,'design');
#36544=PRODUCT_DEFINITION('Bracket_Middle','Bracket_Middle',#36559,#36531);
#36559=PRODUCT_DEFINITION_FORMATION('',$,#36592);
#36578=APPLICATION_CONTEXT(
'Core Data for Automotive Mechanical Design Process');
#36579=PRODUCT_CONTEXT('part definition',#36578,'mechanical');
#36592=PRODUCT('Bracket_Middle','Bracket_Middle',$,(#36579));
#36596=PRESENTATION_STYLE_ASSIGNMENT((#36601));
#36601=SURFACE_STYLE_USAGE(.BOTH.,#36606);
#36606=SURFACE_SIDE_STYLE('',(#36611));
#36611=SURFACE_STYLE_FILL_AREA(#36616);
#36616=FILL_AREA_STYLE('Opaque(160,160,160)',(#36621));
#36621=FILL_AREA_STYLE_COLOUR('Opaque(160,160,160)',#36626);
#36626=COLOUR_RGB('Opaque(160,160,160)', 0.09019608, 0.27058824, 0.51372549);
ENDSEC;
END-ISO-10303-21;
